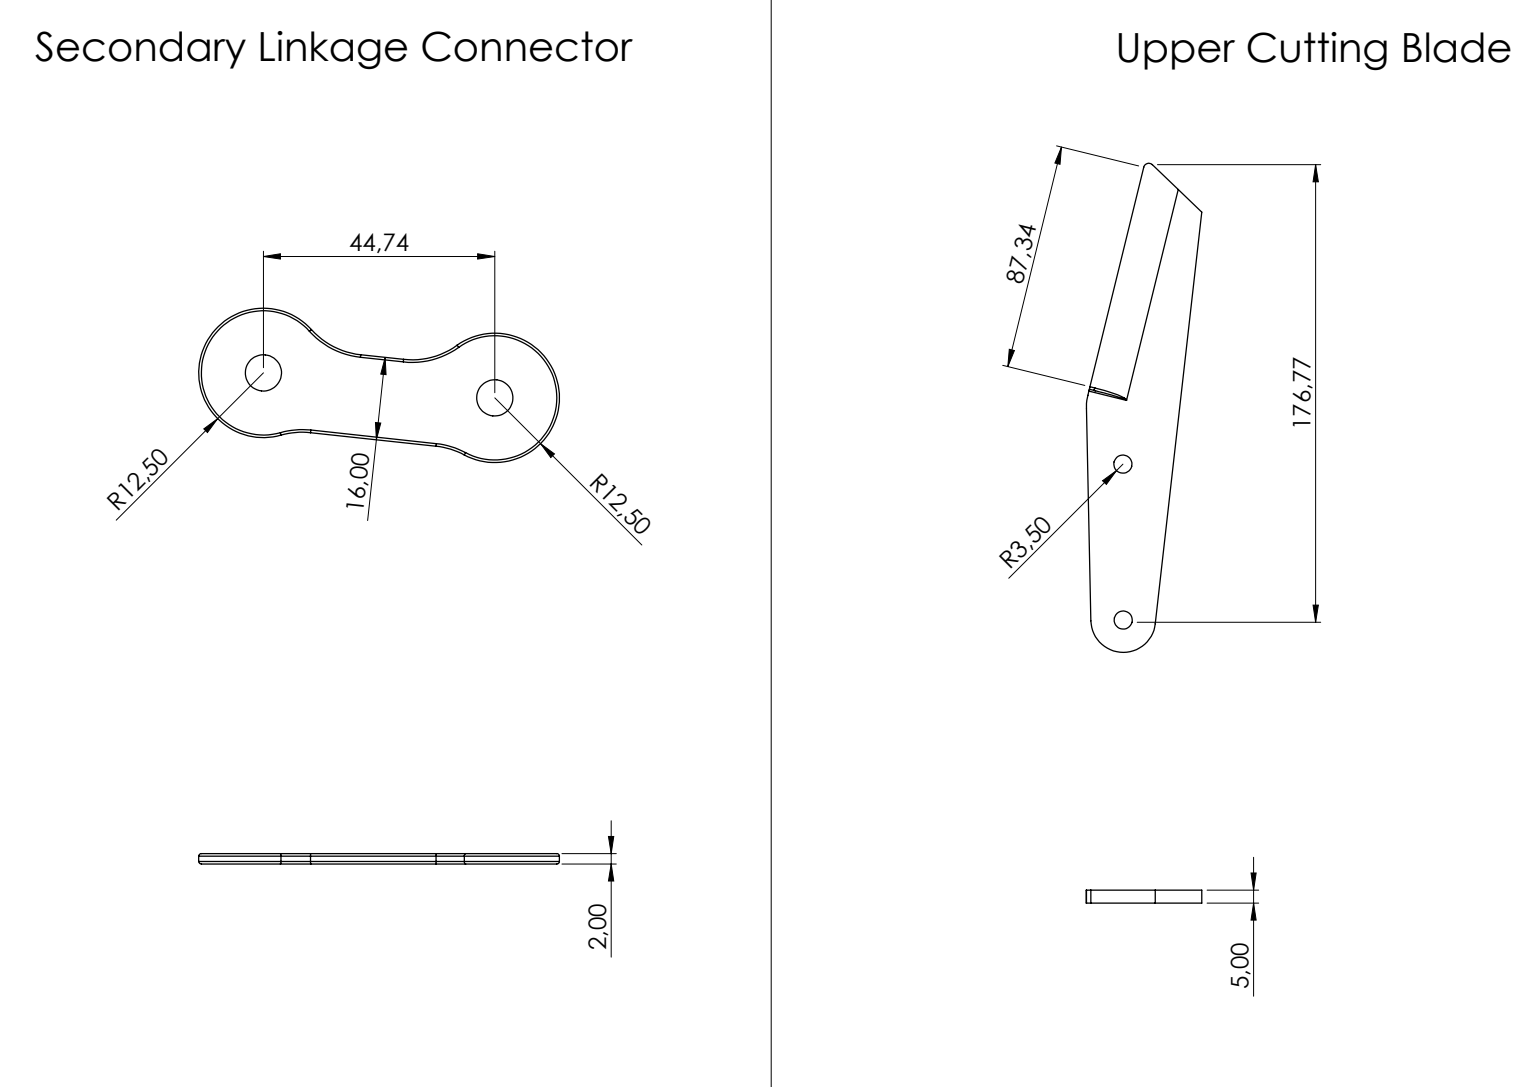
ISO-10303-21;
HEADER;
FILE_DESCRIPTION (('STEP AP214'),
    '1' );
FILE_NAME ('Upper Cutting Blade.step',
    '2026-10-06T08:24:18',
    ( '' ),
    ( '' ),
    'SwSTEP 2.0',
    'SolidWorks 2020',
    '' );
FILE_SCHEMA (( 'AUTOMOTIVE_DESIGN' ));
ENDSEC;

DATA;
#1=B_SPLINE_CURVE_WITH_KNOTS ( 'NONE', 3,
 ( #1947, #5214, #5583, #6285 ),
 .UNSPECIFIED., .F., .F.,
 ( 4, 4 ),
 ( 0.000000000000000000, 1.000000000000000000 ),
 .UNSPECIFIED. ) ;
#2=DIRECTION ( 'NONE',  ( -0.000000000000000000, 1.000000000000000000, 0.000000000000000000 ) ) ;
#8=CARTESIAN_POINT ( 'NONE',  ( -14.98500449093754483, -6.750000000000000000, -438.4247239981262396 ) ) ;
#9=CARTESIAN_POINT ( 'NONE',  ( -1.582652182125599660, -2.660653890702000091, -435.1382991101020821 ) ) ;
#16=CARTESIAN_POINT ( 'NONE',  ( -1.663986357696749074, -7.359447597713999478, -434.8428272099179708 ) ) ;
#37=DIRECTION ( 'NONE',  ( 0.000000000000000000, 1.000000000000000000, 0.000000000000000000 ) ) ;
#44=VECTOR ( 'NONE', #4470, 1000.000000000000114 ) ;
#64=LINE ( 'NONE', #8, #382 ) ;
#71=CARTESIAN_POINT ( 'NONE',  ( -0.1188650835482805701, -7.653137857774001240, -434.2605423690813495 ) ) ;
#78=VERTEX_POINT ( 'NONE', #124 ) ;
#81=CIRCLE ( 'NONE', #4200, 3.500000000000006217 ) ;
#89=CARTESIAN_POINT ( 'NONE',  ( -2.737771089256917811, -7.372713325221263325, -435.0800118814183861 ) ) ;
#97=CARTESIAN_POINT ( 'NONE',  ( -1.873948611767810357, -7.500000000000000000, -349.2478646809746579 ) ) ;
#115=CARTESIAN_POINT ( 'NONE',  ( -11.58158374908019894, -4.051769059165300391, -438.8373653579053553 ) ) ;
#117=DIRECTION ( 'NONE',  ( -0.2381566831044910626, 0.000000000000000000, 0.9712267471052612455 ) ) ;
#119=CARTESIAN_POINT ( 'NONE',  ( -0.6964476799210029823, -2.503143587811580861, -434.2208226102950448 ) ) ;
#124=CARTESIAN_POINT ( 'NONE',  ( -5.273242226636224217, -2.500000000000000000, -350.0814130718403590 ) ) ;
#127=CARTESIAN_POINT ( 'NONE',  ( 8.445486755484310493, -5.763031266960239485, -525.6917925150787596 ) ) ;
#129=CARTESIAN_POINT ( 'NONE',  ( -14.11853184716549059, -5.586257366442001882, -439.2418799830686567 ) ) ;
#131=ORIENTED_EDGE ( 'NONE', *, *, #4319, .T. ) ;
#138=EDGE_CURVE ( 'NONE', #9192, #3634, #10595, .T. ) ;
#140=AXIS2_PLACEMENT_3D ( 'NONE', #9839, #705, #3977 ) ;
#146=VERTEX_POINT ( 'NONE', #9795 ) ;
#152=ADVANCED_FACE ( 'NONE', ( #1627 ), #8180, .F. ) ;
#165=CARTESIAN_POINT ( 'NONE',  ( -3.785374802930533633, -3.175228950698999686, -436.5426513454903557 ) ) ;
#167=CYLINDRICAL_SURFACE ( 'NONE', #9611, 3.500000000000006217 ) ;
#170=CARTESIAN_POINT ( 'NONE',  ( -1.502676399155497666, -2.553500183759497055, -434.6331789313892386 ) ) ;
#174=CARTESIAN_POINT ( 'NONE',  ( -10.10557620461820783, -6.350202160722001388, -437.2724170503247478 ) ) ;
#176=CARTESIAN_POINT ( 'NONE',  ( -0.1242360338837507489, -2.350034431637000765, -434.3027510456794857 ) ) ;
#180=CARTESIAN_POINT ( 'NONE',  ( 8.029177897429777389, -4.293198024933910339, -525.7662775258050942 ) ) ;
#182=CARTESIAN_POINT ( 'NONE',  ( 8.590329508774594558, -5.782842335357056385, -525.6531578069093484 ) ) ;
#191=EDGE_LOOP ( 'NONE', ( #1720, #2254, #5403, #9051 ) ) ;
#202=ORIENTED_EDGE ( 'NONE', *, *, #2410, .F. ) ;
#208=( NAMED_UNIT ( * ) SI_UNIT ( $, .STERADIAN. ) SOLID_ANGLE_UNIT ( ) );
#234=CARTESIAN_POINT ( 'NONE',  ( 7.290921060855201752, -4.384180831252638910, -525.6208113643167508 ) ) ;
#236=CARTESIAN_POINT ( 'NONE',  ( 7.441233258528033190, -5.633901944276541229, -525.6643399796049607 ) ) ;
#238=DIRECTION ( 'NONE',  ( -0.2381557937579781570, -1.220925210680262645E-07, 0.9712269651834695150 ) ) ;
#250=CARTESIAN_POINT ( 'NONE',  ( -2.040571445035855636, -7.414593747479792718, -434.8398329727854730 ) ) ;
#253=EDGE_LOOP ( 'NONE', ( #1986, #2444 ) ) ;
#255=DIRECTION ( 'NONE',  ( -0.000000000000000000, 1.000000000000000000, 0.000000000000000000 ) ) ;
#276=CARTESIAN_POINT ( 'NONE',  ( -0.6583197226283303838, -2.500002886833834204, -434.1455329896276680 ) ) ;
#283=DIRECTION ( 'NONE',  ( -0.000000000000000000, 1.000000000000000000, 0.000000000000000000 ) ) ;
#287=CARTESIAN_POINT ( 'NONE',  ( 28.53863984632670636, -7.500000000000000000, -506.8274460463252353 ) ) ;
#302=DIRECTION ( 'NONE',  ( -0.000000000000000000, 1.000000000000000000, 0.000000000000000000 ) ) ;
#309=EDGE_CURVE ( 'NONE', #4938, #6833, #7633, .T. ) ;
#311=VECTOR ( 'NONE', #7522, 1000.000000000000114 ) ;
#312=B_SPLINE_CURVE_WITH_KNOTS ( 'NONE', 3,
 ( #4614, #3005, #5310, #9407, #7889, #6280, #1335, #5207, #2093, #7044, #1228, #5260, #3810, #10313, #5359, #7836, #485, #2950, #6223, #8534, #8486 ),
 .UNSPECIFIED., .F., .F.,
 ( 4, 1, 1, 1, 2, 2, 1, 1, 1, 1, 1, 1, 2, 2, 4 ),
 ( 0.000000000000000000, 0.2499999999999730771, 0.3749999999999595879, 0.4374999999999530931, 0.4687499999999498734, 0.4999999999999465983, 0.6249999999999374944, 0.6874999999999327205, 0.7187499999999277245, 0.7343749999999221734, 0.7421874999999192868, 0.7460937499999209521, 0.7480468749999217293, 0.7499999999999225064, 1.000000000000000000 ),
 .UNSPECIFIED. ) ;
#313=EDGE_CURVE ( 'NONE', #8716, #4497, #7817, .T. ) ;
#326=LINE ( 'NONE', #4560, #9098 ) ;
#327=DIRECTION ( 'NONE',  ( 0.000000000000000000, -1.000000000000000000, 0.000000000000000000 ) ) ;
#336=CARTESIAN_POINT ( 'NONE',  ( 7.538136778550191153, -5.645663747140947208, -525.6900796742911552 ) ) ;
#342=EDGE_CURVE ( 'NONE', #5251, #8235, #3736, .T. ) ;
#355=DIRECTION ( 'NONE',  ( -0.000000000000000000, 1.000000000000000000, 0.000000000000000000 ) ) ;
#362=CARTESIAN_POINT ( 'NONE',  ( -0.5452757643750816285, -7.478314948056999256, -434.2680375005485871 ) ) ;
#373=EDGE_CURVE ( 'NONE', #5743, #3634, #3350, .T. ) ;
#379=( BOUNDED_SURFACE ( )  B_SPLINE_SURFACE ( 3, 3, ( 
 ( #3396, #9259, #9950, #5161, #8434, #1074, #1023, #5853, #7635, #8489 ),
 ( #9144, #5053, #8334, #972, #4258, #7528, #174, #3449, #9205, #5106 ),
 ( #4309, #3504, #2902, #7046, #4459, #8641, #8536, #5261, #1178, #6121 ),
 ( #7891, #3812, #10155, #4565, #6282, #5361, #3653, #2151, #3007, #7099 ) ),
 .UNSPECIFIED., .F., .F., .T. ) 
 B_SPLINE_SURFACE_WITH_KNOTS ( ( 4, 4 ),
 ( 4, 1, 1, 1, 1, 1, 1, 4 ),
 ( 0.000000000000000000, 1.000000000000000000 ),
 ( 0.04004302100395999708, 0.1036559982346000053, 0.2203786577267000113, 0.3496747522196999580, 0.4912411616719999929, 0.6462853912813000257, 0.8150922079746999449, 0.8736421606905999671 ),
 .UNSPECIFIED. ) 
 GEOMETRIC_REPRESENTATION_ITEM ( )  RATIONAL_B_SPLINE_SURFACE ( (
 ( 1.237064798922000053, 1.237064798922000053, 1.237064798922000053, 1.237064798922000053, 1.237064798922000053, 1.237064798922000053, 1.237064798922000053, 1.237064798922000053, 1.237064798922000053, 1.237064798922000053),
 ( 0.9209784003594999602, 0.9209784003594999602, 0.9209784003594999602, 0.9209784003594999602, 0.9209784003594999602, 0.9209784003594999602, 0.9209784003594999602, 0.9209784003594999602, 0.9209784003594999602, 0.9209784003594999602),
 ( 0.9209784003594999602, 0.9209784003594999602, 0.9209784003594999602, 0.9209784003594999602, 0.9209784003594999602, 0.9209784003594999602, 0.9209784003594999602, 0.9209784003594999602, 0.9209784003594999602, 0.9209784003594999602),
 ( 1.237064798922000053, 1.237064798922000053, 1.237064798922000053, 1.237064798922000053, 1.237064798922000053, 1.237064798922000053, 1.237064798922000053, 1.237064798922000053, 1.237064798922000053, 1.237064798922000053) ) ) 
 REPRESENTATION_ITEM ( '' )  SURFACE ( )  );
#382=VECTOR ( 'NONE', #1674, 1000.000000000000114 ) ;
#385=CARTESIAN_POINT ( 'NONE',  ( 6.150179767644408990, -4.500000000000001776, -524.6161169473078871 ) ) ;
#386=DIRECTION ( 'NONE',  ( 0.9627070496199738869, -0.1321637200910051047, 0.2360675490272045596 ) ) ;
#400=DIRECTION ( 'NONE',  ( -0.9712267471052594692, 0.000000000000000000, -0.2381566831044984178 ) ) ;
#401=ORIENTED_EDGE ( 'NONE', *, *, #4319, .F. ) ;
#407=EDGE_CURVE ( 'NONE', #146, #5498, #4519, .T. ) ;
#409=CARTESIAN_POINT ( 'NONE',  ( -0.7256479603086914976, -7.501867437109999592, -434.1451055704292799 ) ) ;
#418=CARTESIAN_POINT ( 'NONE',  ( -0.6596894340221253206, -7.499999891561000886, -434.1397621899948263 ) ) ;
#429=CARTESIAN_POINT ( 'NONE',  ( -1.582652182125599660, -2.660653890702000091, -435.1382991101020821 ) ) ;
#435=B_SPLINE_CURVE_WITH_KNOTS ( 'NONE', 3,
 ( #4769, #8901, #8094, #8733, #8788, #10403, #10619, #2354, #4014, #790, #6372, #2295 ),
 .UNSPECIFIED., .F., .F.,
 ( 4, 2, 2, 2, 2, 4 ),
 ( 0.000000000000000000, 0.4999999999999995559, 0.7499999999999974465, 0.8749999999999965583, 0.9374999999999983347, 1.000000000000000000 ),
 .UNSPECIFIED. ) ;
#446=CARTESIAN_POINT ( 'NONE',  ( -0.6528312677253685914, -7.479800707286198502, -434.5251259939439024 ) ) ;
#454=CARTESIAN_POINT ( 'NONE',  ( 9.378959784071181360, -5.899999999999999467, -525.1866552614185366 ) ) ;
#464=CARTESIAN_POINT ( 'NONE',  ( -1.658294475769471310, -7.463038962712998270, -434.6370517716558197 ) ) ;
#475=CARTESIAN_POINT ( 'NONE',  ( -1.788249073448326953, -7.429140679109920598, -434.7441729133906279 ) ) ;
#483=DIRECTION ( 'NONE',  ( -0.000000000000000000, 1.000000000000000000, 0.000000000000000000 ) ) ;
#485=CARTESIAN_POINT ( 'NONE',  ( -3.771252382897392952, -2.975477256776445145, -436.1454489244006822 ) ) ;
#501=CARTESIAN_POINT ( 'NONE',  ( -0.5293798494821438938, -2.512522400030999137, -434.0497706731864582 ) ) ;
#519=DIRECTION ( 'NONE',  ( -0.000000000000000000, 1.000000000000000000, 0.000000000000000000 ) ) ;
#521=CARTESIAN_POINT ( 'NONE',  ( -0.9182485701526132971, -7.496877080320997422, -434.3056557713407528 ) ) ;
#526=ORIENTED_EDGE ( 'NONE', *, *, #7256, .F. ) ;
#550=CARTESIAN_POINT ( 'NONE',  ( -1.558284605000191947, -2.631303827346001878, -434.8033654657723446 ) ) ;
#556=DIRECTION ( 'NONE',  ( -0.000000000000000000, 1.000000000000000000, 0.000000000000000000 ) ) ;
#571=CARTESIAN_POINT ( 'NONE',  ( -0.1153702471463786128, -7.665106240334001342, -434.0348060233743581 ) ) ;
#574=VERTEX_POINT ( 'NONE', #5718 ) ;
#583=ORIENTED_EDGE ( 'NONE', *, *, #4956, .T. ) ;
#601=CIRCLE ( 'NONE', #6609, 3.500000000000006217 ) ;
#611=CARTESIAN_POINT ( 'NONE',  ( -1.837389479601686304, -2.655393054924001461, -434.9057872931240354 ) ) ;
#621=DIRECTION ( 'NONE',  ( -0.000000000000000000, 1.000000000000000000, 0.000000000000000000 ) ) ;
#629=CARTESIAN_POINT ( 'NONE',  ( -5.273242226636224217, -7.500000000000000000, -350.0814130718403590 ) ) ;
#637=ADVANCED_FACE ( 'NONE', ( #3830 ), #4049, .F. ) ;
#650=DIRECTION ( 'NONE',  ( -0.000000000000000000, 1.000000000000000000, 0.000000000000000000 ) ) ;
#655=ADVANCED_FACE ( 'NONE', ( #3024 ), #6350, .T. ) ;
#660=CARTESIAN_POINT ( 'NONE',  ( -1.444632214126728043, -2.659134901855999988, -434.9867182716628236 ) ) ;
#664=ORIENTED_EDGE ( 'NONE', *, *, #4434, .T. ) ;
#705=DIRECTION ( 'NONE',  ( -0.9712267471052612455, 0.000000000000000000, -0.2381566831044910626 ) ) ;
#714=CARTESIAN_POINT ( 'NONE',  ( -0.5380925645899466980, -2.513321162497997197, -434.0383604270527940 ) ) ;
#720=FACE_BOUND ( 'NONE', #6913, .T. ) ;
#722=VERTEX_POINT ( 'NONE', #8182 ) ;
#733=CARTESIAN_POINT ( 'NONE',  ( 9.378959784071181360, -5.899999999999999467, -525.1866552614185366 ) ) ;
#748=EDGE_LOOP ( 'NONE', ( #1545, #9667, #1018, #6857 ) ) ;
#752=CARTESIAN_POINT ( 'NONE',  ( -1.999999999997229772, -7.500000000000000000, -409.4999999999571969 ) ) ;
#759=CARTESIAN_POINT ( 'NONE',  ( -3.656057816511529168, -7.040919069177174805, -436.0988728614874503 ) ) ;
#770=EDGE_CURVE ( 'NONE', #2618, #5251, #7738, .T. ) ;
#771=CARTESIAN_POINT ( 'NONE',  ( -1.000888714456147133, -7.421678258158998176, -434.5721179219322039 ) ) ;
#790=CARTESIAN_POINT ( 'NONE',  ( -2.272356604769890431, -2.599354866276060605, -434.9211891149597591 ) ) ;
#805=DIRECTION ( 'NONE',  ( -0.9712267471052594692, 0.000000000000000000, -0.2381566831044984178 ) ) ;
#815=CARTESIAN_POINT ( 'NONE',  ( -15.03660170392436335, -3.530928676948000167, -439.4670019462156461 ) ) ;
#822=CARTESIAN_POINT ( 'NONE',  ( -0.3462645226701464574, -7.523938431909999558, -434.3437067901672322 ) ) ;
#824=CARTESIAN_POINT ( 'NONE',  ( -0.6228901166779408083, -2.499999376604999934, -434.1632067468180480 ) ) ;
#840=ORIENTED_EDGE ( 'NONE', *, *, #770, .T. ) ;
#856=CARTESIAN_POINT ( 'NONE',  ( -13.22841709878402483, -6.750000000003000267, -437.9939892205655383 ) ) ;
#869=CARTESIAN_POINT ( 'NONE',  ( -1.322461528884503412, -7.357049826291000905, -434.9394999171997824 ) ) ;
#880=EDGE_CURVE ( 'NONE', #5498, #146, #2568, .T. ) ;
#890=VERTEX_POINT ( 'NONE', #6702 ) ;
#907=ORIENTED_EDGE ( 'NONE', *, *, #4640, .T. ) ;
#908=CARTESIAN_POINT ( 'NONE',  ( -5.874649674696526880, -3.342435975618997634, -436.3259412683626692 ) ) ;
#922=CARTESIAN_POINT ( 'NONE',  ( -0.9319947458880994962, -7.428963293140000701, -434.5389931698585428 ) ) ;
#943=ORIENTED_EDGE ( 'NONE', *, *, #3912, .F. ) ;
#965=CARTESIAN_POINT ( 'NONE',  ( -11.73517431002995970, -4.202811174509099246, -438.1641048472901616 ) ) ;
#972=CARTESIAN_POINT ( 'NONE',  ( -4.039076881902885496, -6.821318530964001425, -435.8791522177131696 ) ) ;
#979=CARTESIAN_POINT ( 'NONE',  ( 8.820893615063965854, -5.815056166419472206, -525.5682599993908752 ) ) ;
#1002=B_SPLINE_CURVE_WITH_KNOTS ( 'NONE', 3,
 ( #4633, #7160, #7904, #10431, #2110, #3071, #6345, #4521, #7110, #6511, #9846, #5753, #8178, #7372, #9039, #4045, #8278, #2536, #4949, #4849, #2484 ),
 .UNSPECIFIED., .F., .F.,
 ( 4, 1, 1, 1, 2, 2, 2, 2, 1, 1, 2, 2, 4 ),
 ( 0.000000000000000000, 0.1249999999994945710, 0.1874999999991950606, 0.2187499999990910604, 0.2343749999990832888, 0.2499999999990755173, 0.3749999999992109090, 0.4999999999993463007, 0.6249999999994816369, 0.6874999999995808908, 0.7187499999996315170, 0.7499999999996821431, 1.000000000000000000 ),
 .UNSPECIFIED. ) ;
#1005=CARTESIAN_POINT ( 'NONE',  ( -16.11962419174959393, -2.500000000000000000, -430.9361393731155658 ) ) ;
#1014=CARTESIAN_POINT ( 'NONE',  ( -4.040158012961684086, -3.178778163799998779, -435.8794274319448050 ) ) ;
#1018=ORIENTED_EDGE ( 'NONE', *, *, #5034, .F. ) ;
#1022=SURFACE_SIDE_STYLE ('',( #6726 ) ) ;
#1023=CARTESIAN_POINT ( 'NONE',  ( -10.21689005072306422, -7.047891920729001392, -437.2157279943754133 ) ) ;
#1029=CARTESIAN_POINT ( 'NONE',  ( 8.337581009124432896, -4.251569741560065729, -525.7130236167810153 ) ) ;
#1030=CARTESIAN_POINT ( 'NONE',  ( -1.327990674002025528, -7.383908396211002589, -435.1679363805569665 ) ) ;
#1045=( BOUNDED_CURVE ( )  B_SPLINE_CURVE ( 3, ( #9621, #4574, #8700, #6128 ),
 .UNSPECIFIED., .F., .F. ) 
 B_SPLINE_CURVE_WITH_KNOTS ( ( 4, 4 ),
 ( 0.000000000000000000, 1.000000000000000000 ),
 .UNSPECIFIED. ) 
 CURVE ( )  GEOMETRIC_REPRESENTATION_ITEM ( )  RATIONAL_B_SPLINE_CURVE ( ( 1.017160811567055401, 0.9969340269212683125, 0.9945876386442641381, 1.010121646736042766 ) ) 
 REPRESENTATION_ITEM ( '' )  );
#1069=CARTESIAN_POINT ( 'NONE',  ( -1.437615631311345288, -2.692042927306998568, -435.8453383182137486 ) ) ;
#1072=CARTESIAN_POINT ( 'NONE',  ( -0.9894400438770221129, -2.521929977679939316, -434.4064049843834141 ) ) ;
#1074=CARTESIAN_POINT ( 'NONE',  ( -8.039695956235750174, -7.171008361171001155, -436.6144689615417747 ) ) ;
#1088=ORIENTED_EDGE ( 'NONE', *, *, #313, .F. ) ;
#1100=ORIENTED_EDGE ( 'NONE', *, *, #6861, .T. ) ;
#1110=CIRCLE ( 'NONE', #2316, 0.7499999999999997780 ) ;
#1114=CARTESIAN_POINT ( 'NONE',  ( -0.9643324756131976816, -7.495094651894998350, -434.3305354681787662 ) ) ;
#1121=ORIENTED_EDGE ( 'NONE', *, *, #9520, .F. ) ;
#1136=DIRECTION ( 'NONE',  ( 0.000000000000000000, -1.000000000000000000, -0.000000000000000000 ) ) ;
#1139=DIRECTION ( 'NONE',  ( -0.9627072696281171460, 0.1321637200910011078, -0.2360666518102109701 ) ) ;
#1159=B_SPLINE_CURVE_WITH_KNOTS ( 'NONE', 3,
 ( #4416, #8440, #10011, #3561, #979, #5920, #182, #6678, #127, #8392, #9369, #2003, #10113, #9958, #5860, #7693, #7587, #1949, #2753, #336, #4211, #3404, #5115, #3613, #1843, #236, #3456, #5060, #5267, #4370, #9315 ),
 .UNSPECIFIED., .F., .F.,
 ( 4, 2, 2, 2, 1, 1, 1, 2, 2, 2, 2, 1, 1, 1, 1, 2, 2, 2, 4 ),
 ( 0.000000000000000000, 0.1250000000002775280, 0.1875000000004162504, 0.2187500000004856116, 0.2343750000005130896, 0.2421875000005322132, 0.2460937500005417611, 0.2480468750005504208, 0.2500000000005591083, 0.3750000000010509371, 0.4375000000012961299, 0.4687500000014282464, 0.4843750000015074053, 0.4921875000015624169, 0.4960937500015898949, 0.4980468750016032176, 0.5000000000016164847, 0.7500000000008082424, 1.000000000000000000 ),
 .UNSPECIFIED. ) ;
#1163=CARTESIAN_POINT ( 'NONE',  ( -0.8117387980152629412, -7.500462190812000607, -434.2418354198644010 ) ) ;
#1178=CARTESIAN_POINT ( 'NONE',  ( -12.82600522015554922, -5.696851206212700802, -438.3416979569461205 ) ) ;
#1181=FACE_OUTER_BOUND ( 'NONE', #6826, .T. ) ;
#1184=AXIS2_PLACEMENT_3D ( 'NONE', #97, #5779, #6762 ) ;
#1208=CARTESIAN_POINT ( 'NONE',  ( 6.052780067456072999, -4.500000000000000888, -524.2189112390747141 ) ) ;
#1212=FILL_AREA_STYLE_COLOUR ( '', #7652 ) ;
#1222=DIRECTION ( 'NONE',  ( -0.9712267471052611345, 0.000000000000000000, -0.2381566831044912569 ) ) ;
#1228=CARTESIAN_POINT ( 'NONE',  ( -4.443194270446590544, -3.070841006776869886, -436.4083858720387639 ) ) ;
#1236=ORIENTED_EDGE ( 'NONE', *, *, #6395, .F. ) ;
#1238=LINE ( 'NONE', #9569, #7592 ) ;
#1253=ORIENTED_EDGE ( 'NONE', *, *, #1527, .F. ) ;
#1263=ORIENTED_EDGE ( 'NONE', *, *, #3216, .T. ) ;
#1264=STYLED_ITEM ( 'NONE', ( #2643 ), #8937 ) ;
#1274=CARTESIAN_POINT ( 'NONE',  ( -1.249129537600907502, -7.462014900586536825, -434.5271252024986666 ) ) ;
#1291=ADVANCED_FACE ( 'NONE', ( #1181 ), #10221, .T. ) ;
#1300=CARTESIAN_POINT ( 'NONE',  ( -0.6576834034345514501, -2.538582342225996769, -434.3791788602677570 ) ) ;
#1309=CARTESIAN_POINT ( 'NONE',  ( -4.134979495079278422, -6.972766829544778666, -436.2920240787863690 ) ) ;
#1310=CARTESIAN_POINT ( 'NONE',  ( -14.74684780783305449, -4.500000000000000888, -439.3959507452315165 ) ) ;
#1326=B_SPLINE_CURVE_WITH_KNOTS ( 'NONE', 3,
 ( #429, #10262, #8638, #3605 ),
 .UNSPECIFIED., .F., .F.,
 ( 4, 4 ),
 ( 0.000000000000000000, 1.000000000000000000 ),
 .UNSPECIFIED. ) ;
#1332=CARTESIAN_POINT ( 'NONE',  ( 19.38368284813939013, -2.500000000000000000, -515.5999187775453265 ) ) ;
#1335=CARTESIAN_POINT ( 'NONE',  ( -6.619999202174732034, -3.376841163498135234, -437.1676759332182769 ) ) ;
#1338=EDGE_CURVE ( 'NONE', #5915, #6684, #1, .T. ) ;
#1343=CARTESIAN_POINT ( 'NONE',  ( 6.052780067456072999, -4.500000000000000888, -524.2189112390747141 ) ) ;
#1352=CARTESIAN_POINT ( 'NONE',  ( -0.8844900259107285612, -2.565904207356001443, -434.5153608183709935 ) ) ;
#1353=ORIENTED_EDGE ( 'NONE', *, *, #7256, .T. ) ;
#1365=ORIENTED_EDGE ( 'NONE', *, *, #5468, .F. ) ;
#1370=CARTESIAN_POINT ( 'NONE',  ( -1.547234103168566133, -7.369705175477000658, -434.7990518850289163 ) ) ;
#1390=ORIENTED_EDGE ( 'NONE', *, *, #4717, .F. ) ;
#1391=DIRECTION ( 'NONE',  ( -0.9712267471052594692, 0.000000000000000000, -0.2381566831044984178 ) ) ;
#1406=CARTESIAN_POINT ( 'NONE',  ( -0.7175256489034935736, -2.498213111830998923, -434.1510992972750387 ) ) ;
#1419=FACE_OUTER_BOUND ( 'NONE', #4482, .T. ) ;
#1435=CARTESIAN_POINT ( 'NONE',  ( -15.16362200326591569, -7.500000000000000000, -437.6963039377973246 ) ) ;
#1444=CARTESIAN_POINT ( 'NONE',  ( -14.78164251960286890, -4.500000000000000000, -439.2540544344155933 ) ) ;
#1450=CLOSED_SHELL ( 'NONE', ( #6125, #6680, #4249, #152, #2598, #9705, #4681, #8027, #2131, #1291, #655, #6920, #4479, #4185, #3013, #3240, #637, #5572, #6836, #2413, #2799, #2213, #8047, #6176, #7498 ) ) ;
#1454=EDGE_CURVE ( 'NONE', #7492, #9535, #2957, .T. ) ;
#1466=CARTESIAN_POINT ( 'NONE',  ( -0.5984921290374501934, -2.530241314762997629, -434.3301463708660322 ) ) ;
#1473=CARTESIAN_POINT ( 'NONE',  ( -0.5534908175310586653, -2.500000333914000006, -434.2941325283891274 ) ) ;
#1502=CARTESIAN_POINT ( 'NONE',  ( -14.85178883355849599, -4.396734861472281430, -438.9679907580307940 ) ) ;
#1504=ORIENTED_EDGE ( 'NONE', *, *, #2729, .T. ) ;
#1506=PRODUCT_DEFINITION_SHAPE ( 'NONE', 'NONE',  #2191 ) ;
#1518=CARTESIAN_POINT ( 'NONE',  ( -1.668977462971013681, -2.537472099014000726, -434.6413441610087034 ) ) ;
#1521=DIRECTION ( 'NONE',  ( -0.000000000000000000, 1.000000000000000000, 0.000000000000000000 ) ) ;
#1527=EDGE_CURVE ( 'NONE', #9271, #890, #5926, .T. ) ;
#1528=EDGE_LOOP ( 'NONE', ( #5275, #7312, #1559, #3644, #3139, #4760, #5881, #4377, #9229 ) ) ;
#1530=VERTEX_POINT ( 'NONE', #5273 ) ;
#1545=ORIENTED_EDGE ( 'NONE', *, *, #9391, .T. ) ;
#1559=ORIENTED_EDGE ( 'NONE', *, *, #4277, .T. ) ;
#1576=CARTESIAN_POINT ( 'NONE',  ( -0.1454145850583489497, -8.513384478312998382, -435.8155006440865691 ) ) ;
#1580=CARTESIAN_POINT ( 'NONE',  ( -0.4619277171041915042, -7.556499546952999857, -434.7365042083650906 ) ) ;
#1582=DIRECTION ( 'NONE',  ( -0.9712267471052612455, 0.000000000000000000, -0.2381566831044910626 ) ) ;
#1583=FACE_OUTER_BOUND ( 'NONE', #10228, .T. ) ;
#1592=AXIS2_PLACEMENT_3D ( 'NONE', #4702, #621, #6470 ) ;
#1599=ORIENTED_EDGE ( 'NONE', *, *, #3133, .T. ) ;
#1626=CARTESIAN_POINT ( 'NONE',  ( -1.486103177728019809, -2.642483842335999089, -435.2287432255328667 ) ) ;
#1627=FACE_OUTER_BOUND ( 'NONE', #4357, .T. ) ;
#1633=CARTESIAN_POINT ( 'NONE',  ( -0.5253760780244931539, -7.541458695310001126, -434.7805624543377689 ) ) ;
#1639=ORIENTED_EDGE ( 'NONE', *, *, #5745, .F. ) ;
#1644=DIRECTION ( 'NONE',  ( 0.9936574763089274231, 0.000000000000000000, 0.1124491875265153373 ) ) ;
#1663=ORIENTED_EDGE ( 'NONE', *, *, #407, .T. ) ;
#1674=DIRECTION ( 'NONE',  ( 0.9712269959794516128, -1.472254293302932272E-12, 0.2381556681683856258 ) ) ;
#1682=EDGE_CURVE ( 'NONE', #9271, #722, #5114, .T. ) ;
#1683=CARTESIAN_POINT ( 'NONE',  ( -0.1066158053962373981, -7.660711547938000798, -434.1593156514779253 ) ) ;
#1696=PLANE ( 'NONE',  #3521 ) ;
#1720=ORIENTED_EDGE ( 'NONE', *, *, #1454, .F. ) ;
#1722=CARTESIAN_POINT ( 'NONE',  ( -1.723815153757401353, -2.911508528774001459, -435.2348705281305001 ) ) ;
#1728=CARTESIAN_POINT ( 'NONE',  ( -0.6577138333327989805, -2.500183709831155454, -434.1612907480973149 ) ) ;
#1735=CARTESIAN_POINT ( 'NONE',  ( -1.121771287418490415, -7.384865809656000479, -434.8579640789354244 ) ) ;
#1748=CARTESIAN_POINT ( 'NONE',  ( -1.813125098999968543, -7.427867185880000278, -434.7536662776001322 ) ) ;
#1754=ORIENTED_EDGE ( 'NONE', *, *, #3459, .T. ) ;
#1759=EDGE_CURVE ( 'NONE', #6366, #4799, #1002, .T. ) ;
#1760=LINE ( 'NONE', #9929, #4624 ) ;
#1775=FACE_OUTER_BOUND ( 'NONE', #748, .T. ) ;
#1780=CARTESIAN_POINT ( 'NONE',  ( -0.6695406252879771980, -2.501212138556309306, -434.1886289273209627 ) ) ;
#1785=CARTESIAN_POINT ( 'NONE',  ( -0.1791381520249625270, -2.339610688496001512, -433.8702690752436411 ) ) ;
#1790=CARTESIAN_POINT ( 'NONE',  ( -1.009071087474297190, -7.440846336948001571, -435.0353261705186583 ) ) ;
#1803=DIRECTION ( 'NONE',  ( -0.000000000000000000, 1.000000000000000000, 0.000000000000000000 ) ) ;
#1821=( NAMED_UNIT ( * ) PLANE_ANGLE_UNIT ( ) SI_UNIT ( $, .RADIAN. ) );
#1833=LINE ( 'NONE', #856, #311 ) ;
#1842=CARTESIAN_POINT ( 'NONE',  ( 9.378959784071181360, -4.100000000000000533, -525.1866552614185366 ) ) ;
#1843=CARTESIAN_POINT ( 'NONE',  ( 7.441755802380456863, -5.633964924930761065, -525.6644890118283229 ) ) ;
#1870=EDGE_LOOP ( 'NONE', ( #10144, #6393 ) ) ;
#1882=CARTESIAN_POINT ( 'NONE',  ( -12.67186291068377102, -4.210876960398400648, -439.0233713709748145 ) ) ;
#1886=CIRCLE ( 'NONE', #4802, 1.000010080120980804 ) ;
#1896=CARTESIAN_POINT ( 'NONE',  ( 6.760923308610696125, -4.443194654328453730, -525.3178833974152440 ) ) ;
#1898=CARTESIAN_POINT ( 'NONE',  ( -12.86189863199293093, -5.758762107780500017, -438.9337381413729418 ) ) ;
#1917=FACE_OUTER_BOUND ( 'NONE', #7814, .T. ) ;
#1927=LINE ( 'NONE', #7567, #7093 ) ;
#1936=CARTESIAN_POINT ( 'NONE',  ( -13.08309215884270138, -3.120241701627000985, -437.9645355315274173 ) ) ;
#1941=( NAMED_UNIT ( * ) PLANE_ANGLE_UNIT ( ) SI_UNIT ( $, .RADIAN. ) );
#1947=CARTESIAN_POINT ( 'NONE',  ( -1.813125407131493949, -2.572135581867000198, -434.7536649739391237 ) ) ;
#1948=FACE_BOUND ( 'NONE', #10054, .T. ) ;
#1949=CARTESIAN_POINT ( 'NONE',  ( 7.681427628432651922, -5.663384406618502176, -525.7189183918870867 ) ) ;
#1952=EDGE_CURVE ( 'NONE', #8193, #5743, #2223, .T. ) ;
#1957=ORIENTED_EDGE ( 'NONE', *, *, #4434, .F. ) ;
#1968=CYLINDRICAL_SURFACE ( 'NONE', #9194, 0.7499999999999997780 ) ;
#1977=CARTESIAN_POINT ( 'NONE',  ( -0.5023555725018206131, -7.489090630217000388, -434.1119911457818716 ) ) ;
#1985=LINE ( 'NONE', #2188, #10502 ) ;
#1986=ORIENTED_EDGE ( 'NONE', *, *, #3319, .T. ) ;
#1987=CARTESIAN_POINT ( 'NONE',  ( -0.6780083913994491285, -7.498182470000450017, -434.1985855385974560 ) ) ;
#2003=CARTESIAN_POINT ( 'NONE',  ( 8.342417508530179049, -5.749081105070941611, -525.7122382318706286 ) ) ;
#2009=DIRECTION ( 'NONE',  ( 0.2381566831044910626, 0.000000000000000000, -0.9712267471052612455 ) ) ;
#2019=ORIENTED_EDGE ( 'NONE', *, *, #4921, .T. ) ;
#2025=CARTESIAN_POINT ( 'NONE',  ( -1.873948611767810357, -7.500000000000000000, -349.2478646809746579 ) ) ;
#2027=CARTESIAN_POINT ( 'NONE',  ( -0.5174164570134516250, -7.488494838810996868, -434.0682185966899169 ) ) ;
#2032=ORIENTED_EDGE ( 'NONE', *, *, #3049, .T. ) ;
#2057=LINE ( 'NONE', #6086, #10332 ) ;
#2071=DIRECTION ( 'NONE',  ( 0.6918631112021627061, 0.000000000000000000, -0.7220286942758327164 ) ) ;
#2076=CARTESIAN_POINT ( 'NONE',  ( -0.7865748771364371450, -7.501119061185001158, -434.2245970632208127 ) ) ;
#2087=CARTESIAN_POINT ( 'NONE',  ( -15.34933947562448076, -6.750000000000000000, -437.7418441346085274 ) ) ;
#2093=CARTESIAN_POINT ( 'NONE',  ( -5.875275055693564674, -3.272594625989450723, -436.9218166935183376 ) ) ;
#2099=DIRECTION ( 'NONE',  ( -0.2381566831044918675, 0.000000000000000000, 0.9712267471052610235 ) ) ;
#2110=CARTESIAN_POINT ( 'NONE',  ( -14.83150119643293330, -5.565240525586856002, -439.0507257690958909 ) ) ;
#2112=ORIENTED_EDGE ( 'NONE', *, *, #2260, .T. ) ;
#2129=MECHANICAL_DESIGN_GEOMETRIC_PRESENTATION_REPRESENTATION('',(#1264),#10532);
#2130=CARTESIAN_POINT ( 'NONE',  ( -1.284201520726217627, -7.481087858561002335, -434.4823192484363403 ) ) ;
#2131=ADVANCED_FACE ( 'NONE', ( #8935 ), #5707, .T. ) ;
#2151=CARTESIAN_POINT ( 'NONE',  ( -11.57898025333339831, -5.948622255021098759, -438.8369007677023319 ) ) ;
#2165=CARTESIAN_POINT ( 'NONE',  ( -0.4139159552628927652, -2.492503281179000663, -434.4399094585419903 ) ) ;
#2181=CARTESIAN_POINT ( 'NONE',  ( -1.552911365449734626, -7.327055393686999984, -435.0269566445958276 ) ) ;
#2188=CARTESIAN_POINT ( 'NONE',  ( -14.98500449093754483, -6.508849730028000380, -438.4247239981262396 ) ) ;
#2190=CARTESIAN_POINT ( 'NONE',  ( -1.099124599181354522, -7.471261185735560417, -434.4594340131810100 ) ) ;
#2191=PRODUCT_DEFINITION ( 'UNKNOWN', '', #5412, #7223 ) ;
#2213=ADVANCED_FACE ( 'NONE', ( #1948, #9905, #2651 ), #3510, .T. ) ;
#2218=CARTESIAN_POINT ( 'NONE',  ( -0.3413170418743253776, -2.457820343117000039, -433.9546262319294669 ) ) ;
#2223=LINE ( 'NONE', #6352, #6367 ) ;
#2241=ORIENTED_EDGE ( 'NONE', *, *, #6861, .F. ) ;
#2254=ORIENTED_EDGE ( 'NONE', *, *, #9718, .F. ) ;
#2260=EDGE_CURVE ( 'NONE', #5868, #10390, #7313, .T. ) ;
#2270=CARTESIAN_POINT ( 'NONE',  ( -1.170915164613087756, -2.622174536531001188, -434.8787092738958791 ) ) ;
#2274=ORIENTED_EDGE ( 'NONE', *, *, #5034, .T. ) ;
#2278=UNCERTAINTY_MEASURE_WITH_UNIT (LENGTH_MEASURE( 1.000000000000000082E-05 ), #10040, 'distance_accuracy_value', 'NONE');
#2295=CARTESIAN_POINT ( 'NONE',  ( -1.813125407131493949, -2.572135581867000198, -434.7536649739391237 ) ) ;
#2304=CARTESIAN_POINT ( 'NONE',  ( -15.54870946350325767, -7.500000000000000000, -436.1258788022018393 ) ) ;
#2315=CYLINDRICAL_SURFACE ( 'NONE', #3737, 3.500000000000006217 ) ;
#2316=AXIS2_PLACEMENT_3D ( 'NONE', #7503, #9874, #37 ) ;
#2326=CARTESIAN_POINT ( 'NONE',  ( -1.897969053490322855, -2.548986172702000896, -434.7293254325074940 ) ) ;
#2333=VERTEX_POINT ( 'NONE', #2805 ) ;
#2345=B_SPLINE_CURVE_WITH_KNOTS ( 'NONE', 3,
 ( #1748, #250, #9010, #89, #8197, #5824, #3366, #6643, #9918, #2555, #9116, #10178 ),
 .UNSPECIFIED., .F., .F.,
 ( 4, 2, 2, 2, 2, 4 ),
 ( 0.000000000000000000, 0.06249999999999888978, 0.1249999999999977796, 0.2499999999999998890, 0.4999999999999998890, 1.000000000000000000 ),
 .UNSPECIFIED. ) ;
#2354=CARTESIAN_POINT ( 'NONE',  ( -2.971092673426039443, -2.641283117323076191, -435.1576634133632524 ) ) ;
#2364=B_SPLINE_CURVE_WITH_KNOTS ( 'NONE', 3,
 ( #8051, #7252, #5630, #3921, #3869, #8746, #5578, #4027, #4081, #8860, #7146, #10579, #10520, #1502, #4784, #3222, #1444, #6384 ),
 .UNSPECIFIED., .F., .F.,
 ( 4, 1, 1, 1, 1, 2, 2, 1, 1, 2, 2, 4 ),
 ( 0.000000000000000000, 0.2499999999994746425, 0.3749999999992318367, 0.4374999999991385780, 0.4687499999990925592, 0.4843749999990695221, 0.4999999999990465405, 0.6249999999991870947, 0.6874999999993030020, 0.7187499999993127719, 0.7499999999993226529, 1.000000000000000000 ),
 .UNSPECIFIED. ) ;
#2367=CARTESIAN_POINT ( 'NONE',  ( -1.873948611767810357, -2.500000000000000000, -349.2478646809746579 ) ) ;
#2378=CARTESIAN_POINT ( 'NONE',  ( -2.975649281827347448, -7.138022370016234852, -435.8156820327864693 ) ) ;
#2380=CARTESIAN_POINT ( 'NONE',  ( -0.8018440996563184209, -2.556536707011997311, -434.4710415144371041 ) ) ;
#2385=CARTESIAN_POINT ( 'NONE',  ( -0.3206729354815163191, -7.530925261025000594, -434.2912207255791373 ) ) ;
#2393=ORIENTED_EDGE ( 'NONE', *, *, #3216, .F. ) ;
#2410=EDGE_CURVE ( 'NONE', #4588, #6311, #9403, .T. ) ;
#2413=ADVANCED_FACE ( 'NONE', ( #6394 ), #2315, .F. ) ;
#2429=CARTESIAN_POINT ( 'NONE',  ( -3.355145859302810507, -7.083804960661745476, -435.9754648412450138 ) ) ;
#2438=CARTESIAN_POINT ( 'NONE',  ( -0.1525530514593775588, -7.663337276471000159, -433.9190241679935411 ) ) ;
#2440=CARTESIAN_POINT ( 'NONE',  ( -0.5691333845031163463, -2.499999797932000334, -434.2421446687361026 ) ) ;
#2444=ORIENTED_EDGE ( 'NONE', *, *, #9718, .T. ) ;
#2450=FACE_OUTER_BOUND ( 'NONE', #7648, .T. ) ;
#2468=FACE_OUTER_BOUND ( 'NONE', #6148, .T. ) ;
#2484=CARTESIAN_POINT ( 'NONE',  ( -14.98500449093754483, -6.508849730028000380, -438.4247239981262396 ) ) ;
#2490=VECTOR ( 'NONE', #4188, 1000.000000000000000 ) ;
#2494=CARTESIAN_POINT ( 'NONE',  ( -1.219008076252173778, -7.371161895518000939, -434.8982261995575413 ) ) ;
#2528=CARTESIAN_POINT ( 'NONE',  ( -2.038789940206844342, -2.521785824191000280, -434.7311834052255790 ) ) ;
#2532=CARTESIAN_POINT ( 'NONE',  ( -1.743229001746446682, -2.568129413088056978, -434.7271494043006896 ) ) ;
#2536=CARTESIAN_POINT ( 'NONE',  ( -14.96226901326146042, -6.078566365972378982, -438.5174415475119076 ) ) ;
#2537=CARTESIAN_POINT ( 'NONE',  ( -0.5141583095772008782, -2.456010981267997551, -434.7739004999450003 ) ) ;
#2541=CARTESIAN_POINT ( 'NONE',  ( 8.369319885711609786, -4.247274070869474727, -525.7071792109185253 ) ) ;
#2543=CARTESIAN_POINT ( 'NONE',  ( -1.730441907225505727, -7.305146192242999881, -435.0908526137575905 ) ) ;
#2555=CARTESIAN_POINT ( 'NONE',  ( -9.379641673262440804, -6.977332597345990095, -437.0255175026235293 ) ) ;
#2558=ORIENTED_EDGE ( 'NONE', *, *, #4956, .F. ) ;
#2559=CARTESIAN_POINT ( 'NONE',  ( -0.6233307549567066452, -7.499999885133000532, -434.1629327817910280 ) ) ;
#2568=CIRCLE ( 'NONE', #1184, 3.500000000000006217 ) ;
#2581=( BOUNDED_CURVE ( )  B_SPLINE_CURVE ( 3, ( #7578, #9947, #2532, #7421, #170, #5965, #6014, #8332, #9091, #1072, #2642, #3447, #10002, #4358, #119, #1780, #1728, #276, #8222 ),
 .UNSPECIFIED., .F., .T. ) 
 B_SPLINE_CURVE_WITH_KNOTS ( ( 4, 1, 1, 1, 1, 1, 1, 1, 1, 1, 1, 1, 1, 1, 1, 1, 4 ),
 ( 0.000000000000000000, 0.02240047936246757077, 0.1327950495784611662, 0.2340085511830341525, 0.3267384236920149454, 0.4118026492331378074, 0.4900892306436237522, 0.5625168287438816472, 0.6299155825606346237, 0.6928641569844152803, 0.7516748739333113383, 0.8063000023450603848, 0.8556381163399817691, 0.8990751865928527931, 0.9381911258101325313, 0.9762570717716427815, 1.000000000000000000 ),
 .UNSPECIFIED. ) 
 CURVE ( )  GEOMETRIC_REPRESENTATION_ITEM ( )  RATIONAL_B_SPLINE_CURVE ( ( 1.017164269003578481, 1.017164269003578481, 1.017164269003578481, 1.017164269003578481, 1.017164269003578481, 1.017164269003578481, 1.017164269003578481, 1.017164269003578481, 1.017164269003578481, 1.017164269003578481, 1.017164269003578481, 1.017164269003578481, 1.017164269003578481, 1.017164269003578481, 1.017164269003578481, 1.017164269003578481, 1.017164269003578481, 1.017164269003578481, 1.017164269003578481 ) ) 
 REPRESENTATION_ITEM ( '' )  );
#2582=CARTESIAN_POINT ( 'NONE',  ( -1.093371887104504614, -1.934387371788998111, -435.9299591300448924 ) ) ;
#2596=EDGE_CURVE ( 'NONE', #9045, #4799, #1833, .T. ) ;
#2597=CARTESIAN_POINT ( 'NONE',  ( 7.733184489064065303, -4.330975896438657102, -525.7488827635337429 ) ) ;
#2598=ADVANCED_FACE ( 'NONE', ( #1775 ), #6545, .F. ) ;
#2601=CARTESIAN_POINT ( 'NONE',  ( -12.99025672594594027, -3.249999999996000088, -438.9652310147267826 ) ) ;
#2618=VERTEX_POINT ( 'NONE', #6777 ) ;
#2619=CIRCLE ( 'NONE', #6036, 20.00000000000000355 ) ;
#2628=AXIS2_PLACEMENT_3D ( 'NONE', #7742, #6231, #386 ) ;
#2637=CARTESIAN_POINT ( 'NONE',  ( -7.895874901503558085, -3.499933318827000317, -436.7910735983360269 ) ) ;
#2642=CARTESIAN_POINT ( 'NONE',  ( -0.9130074951844157072, -2.517145578169100339, -434.3665436561622641 ) ) ;
#2643=PRESENTATION_STYLE_ASSIGNMENT (( #6621 ) ) ;
#2651=FACE_OUTER_BOUND ( 'NONE', #1528, .T. ) ;
#2652=CARTESIAN_POINT ( 'NONE',  ( -1.630004931178638428, -7.334531690290998718, -435.2814510150427054 ) ) ;
#2656=ORIENTED_EDGE ( 'NONE', *, *, #4640, .F. ) ;
#2660=CARTESIAN_POINT ( 'NONE',  ( -14.74684780783305449, -5.500000000000000000, -439.3959507452315165 ) ) ;
#2682=( NAMED_UNIT ( * ) SI_UNIT ( $, .STERADIAN. ) SOLID_ANGLE_UNIT ( ) );
#2722=DIRECTION ( 'NONE',  ( 0.000000000000000000, 1.000000000000000000, 0.000000000000000000 ) ) ;
#2725=CARTESIAN_POINT ( 'NONE',  ( 7.995233561666595712, -7.656480000000000175, -523.7425978728656446 ) ) ;
#2729=EDGE_CURVE ( 'NONE', #5743, #4172, #6115, .T. ) ;
#2730=CARTESIAN_POINT ( 'NONE',  ( -1.867120547373915418, -7.452566320787000542, -434.7177009740820495 ) ) ;
#2737=EDGE_LOOP ( 'NONE', ( #9055, #9053, #1639, #5609, #7501 ) ) ;
#2742=CARTESIAN_POINT ( 'NONE',  ( -1.119552414421413511, -2.606163259540000610, -435.7158780125686235 ) ) ;
#2745=AXIS2_PLACEMENT_3D ( 'NONE', #2601, #7695, #3405 ) ;
#2752=CARTESIAN_POINT ( 'NONE',  ( 6.685859146470366277, -4.450907801408272135, -525.2546656924790796 ) ) ;
#2753=CARTESIAN_POINT ( 'NONE',  ( 7.584651611965206541, -5.651391369166294254, -525.7002755026068144 ) ) ;
#2755=ORIENTED_EDGE ( 'NONE', *, *, #8377, .T. ) ;
#2765=DIRECTION ( 'NONE',  ( -0.9712267471052594692, 0.000000000000000000, -0.2381566831044984178 ) ) ;
#2771=DIRECTION ( 'NONE',  ( -0.9712267471052612455, 0.000000000000000000, -0.2381566831044910626 ) ) ;
#2779=CARTESIAN_POINT ( 'NONE',  ( -0.5013770514288425906, -7.487604982435999368, -434.1602016854106978 ) ) ;
#2780=SHAPE_REPRESENTATION_RELATIONSHIP ( 'NONE' , 'NONE' ,  #4085, #5834 ) ;
#2798=CARTESIAN_POINT ( 'NONE',  ( 3.875825478601963248, -7.500000000000000000, -431.3627451401119970 ) ) ;
#2799=ADVANCED_FACE ( 'NONE', ( #6064 ), #7094, .F. ) ;
#2805=CARTESIAN_POINT ( 'NONE',  ( -12.86189863199293093, -5.758762107780500017, -438.9337381413729418 ) ) ;
#2806=CARTESIAN_POINT ( 'NONE',  ( -1.214899924133375331, -7.403467476614999043, -435.1227120718077686 ) ) ;
#2817=AXIS2_PLACEMENT_3D ( 'NONE', #8634, #3966, #3161 ) ;
#2837=AXIS2_PLACEMENT_3D ( 'NONE', #8842, #5662, #10447 ) ;
#2838=CARTESIAN_POINT ( 'NONE',  ( -1.207139762621110890, -7.484635725423999908, -434.4480596911860175 ) ) ;
#2844=CARTESIAN_POINT ( 'NONE',  ( -0.7342372444761647854, -7.494317894969175775, -434.2532513144291215 ) ) ;
#2856=CARTESIAN_POINT ( 'NONE',  ( 3.875825478601963248, -7.656480000000000175, -431.3627451401119970 ) ) ;
#2892=CARTESIAN_POINT ( 'NONE',  ( -0.6592970117152722187, -7.499999799589161853, -434.1413533491637509 ) ) ;
#2902=CARTESIAN_POINT ( 'NONE',  ( -2.301302514452984394, -7.114149834682999440, -436.1192177104634879 ) ) ;
#2925=VERTEX_POINT ( 'NONE', #10248 ) ;
#2930=ORIENTED_EDGE ( 'NONE', *, *, #407, .F. ) ;
#2943=DIRECTION ( 'NONE',  ( 0.000000000000000000, -1.000000000000000000, 0.000000000000000000 ) ) ;
#2950=CARTESIAN_POINT ( 'NONE',  ( -3.766936453924772277, -2.974863205562146007, -436.1437120911318743 ) ) ;
#2952=CARTESIAN_POINT ( 'NONE',  ( -1.999999999997229772, -2.500000000000000000, -409.4999999999571969 ) ) ;
#2957=LINE ( 'NONE', #6997, #6598 ) ;
#2961=FACE_OUTER_BOUND ( 'NONE', #7228, .T. ) ;
#2968=CARTESIAN_POINT ( 'NONE',  ( -0.8331085234012651775, -2.500134501855002078, -434.2559579827629364 ) ) ;
#2983=DIRECTION ( 'NONE',  ( -0.1124491875265152124, 0.000000000000000000, 0.9936574763089273121 ) ) ;
#2986=CARTESIAN_POINT ( 'NONE',  ( -0.6600535743662629962, -7.458390606629000885, -434.6313374073768614 ) ) ;
#2995=CARTESIAN_POINT ( 'NONE',  ( -1.333798302234134647, -7.456821208003824530, -434.5634752832991694 ) ) ;
#2999=CARTESIAN_POINT ( 'NONE',  ( -1.999999999997229772, -7.500000000000000000, -409.4999999999571969 ) ) ;
#3005=CARTESIAN_POINT ( 'NONE',  ( -11.69802267049820976, -4.081445891925754133, -438.6483114700716897 ) ) ;
#3007=CARTESIAN_POINT ( 'NONE',  ( -12.67039042656561243, -5.789333632204900937, -439.0231271474323762 ) ) ;
#3011=CARTESIAN_POINT ( 'NONE',  ( 6.353028986609323248, -4.484463380032637225, -524.9540790665465693 ) ) ;
#3013=ADVANCED_FACE ( 'NONE', ( #3690 ), #5514, .F. ) ;
#3020=CARTESIAN_POINT ( 'NONE',  ( -0.8897543176725906111, -2.502046059794002186, -434.2898615358246843 ) ) ;
#3024=FACE_OUTER_BOUND ( 'NONE', #5286, .T. ) ;
#3028=AXIS2_PLACEMENT_3D ( 'NONE', #2856, #8539, #5971 ) ;
#3040=ORIENTED_EDGE ( 'NONE', *, *, #9427, .F. ) ;
#3049=EDGE_CURVE ( 'NONE', #4096, #4227, #1159, .T. ) ;
#3063=EDGE_CURVE ( 'NONE', #9535, #4497, #8204, .T. ) ;
#3065=DIRECTION ( 'NONE',  ( -0.2381566831044910626, 0.000000000000000000, 0.9712267471052612455 ) ) ;
#3071=CARTESIAN_POINT ( 'NONE',  ( -14.83733877544362478, -5.575412435490171070, -439.0269195386780439 ) ) ;
#3072=CARTESIAN_POINT ( 'NONE',  ( -1.729952635784063331, -2.694803404275001313, -435.0907047969546966 ) ) ;
#3075=DIRECTION ( 'NONE',  ( -0.2381566831044917565, 0.000000000000000000, 0.9712267471052610235 ) ) ;
#3080=ORIENTED_EDGE ( 'NONE', *, *, #3319, .F. ) ;
#3107=CARTESIAN_POINT ( 'NONE',  ( 19.38368284813939013, -7.500000000000000000, -515.5999187775453265 ) ) ;
#3111=CARTESIAN_POINT ( 'NONE',  ( 28.53863984632670636, -2.500000000000000000, -506.8274460463252353 ) ) ;
#3126=CARTESIAN_POINT ( 'NONE',  ( -0.7288599747256179207, -2.498024261830999571, -434.1773087478343314 ) ) ;
#3133=EDGE_CURVE ( 'NONE', #10390, #9641, #5424, .T. ) ;
#3139=ORIENTED_EDGE ( 'NONE', *, *, #309, .T. ) ;
#3147=LINE ( 'NONE', #733, #9358 ) ;
#3149=EDGE_CURVE ( 'NONE', #574, #722, #1045, .T. ) ;
#3159=COLOUR_RGB ( '', 0.66274510, 0.83137255, 0.94901961) ;
#3161=DIRECTION ( 'NONE',  ( 1.000000000000000000, 0.000000000000000000, 0.000000000000000000 ) ) ;
#3165=LINE ( 'NONE', #3107, #6217 ) ;
#3184=CARTESIAN_POINT ( 'NONE',  ( -0.7166823250270980550, -2.498181146152001819, -434.1608823843793061 ) ) ;
#3188=STYLED_ITEM ( 'NONE', ( #7767 ), #5834 ) ;
#3191=CARTESIAN_POINT ( 'NONE',  ( -0.2949131312215419465, -7.545445293999001990, -434.0704074631209437 ) ) ;
#3195=CARTESIAN_POINT ( 'NONE',  ( -0.5535498271043974849, -7.499999952522999891, -434.2938920418101816 ) ) ;
#3203=DIRECTION ( 'NONE',  ( -0.000000000000000000, 1.000000000000000000, 0.000000000000000000 ) ) ;
#3216=EDGE_CURVE ( 'NONE', #146, #2925, #1238, .T. ) ;
#3222=CARTESIAN_POINT ( 'NONE',  ( -14.81438263496213814, -4.470068862813207922, -439.1205369730296297 ) ) ;
#3233=CARTESIAN_POINT ( 'NONE',  ( -3.707567269721498526, -7.033586184390685503, -436.1197384410193081 ) ) ;
#3236=CARTESIAN_POINT ( 'NONE',  ( -0.9356534891085935834, -2.545231261524000033, -435.0024077940244638 ) ) ;
#3237=CARTESIAN_POINT ( 'NONE',  ( -14.37110465573396212, -2.500000000000000000, -348.9812360766022721 ) ) ;
#3240=ADVANCED_FACE ( 'NONE', ( #2961 ), #6950, .F. ) ;
#3242=CARTESIAN_POINT ( 'NONE',  ( -1.837856579518353906, -7.344572662436001487, -434.9059567300546973 ) ) ;
#3277=CARTESIAN_POINT ( 'NONE',  ( -15.54870946350325767, -2.500000000000000000, -436.1258788022018393 ) ) ;
#3282=CARTESIAN_POINT ( 'NONE',  ( -5.399293614865643853, -7.500000000000000000, -410.3335483908228980 ) ) ;
#3283=CARTESIAN_POINT ( 'NONE',  ( -8.369756866907680504, -6.378185918057877934, -437.7466453813695466 ) ) ;
#3291=CARTESIAN_POINT ( 'NONE',  ( -0.7231407225213108969, -7.447240517548999961, -434.6679473676751400 ) ) ;
#3293=CARTESIAN_POINT ( 'NONE',  ( -16.17578790646000186, -2.500000000000000000, -433.5685902625999688 ) ) ;
#3295=ORIENTED_EDGE ( 'NONE', *, *, #8906, .F. ) ;
#3319=EDGE_CURVE ( 'NONE', #7492, #8716, #5526, .T. ) ;
#3334=CARTESIAN_POINT ( 'NONE',  ( -9.899579175599695802, -4.014440445723298723, -437.8439261505764648 ) ) ;
#3336=VECTOR ( 'NONE', #6671, 1000.000000000000000 ) ;
#3348=CIRCLE ( 'NONE', #5540, 3.500000000000005773 ) ;
#3350=CIRCLE ( 'NONE', #2837, 19.99999999999999289 ) ;
#3353=CARTESIAN_POINT ( 'NONE',  ( -0.3768446329310572995, -7.516309540199999084, -434.3911927895006784 ) ) ;
#3366=CARTESIAN_POINT ( 'NONE',  ( -4.143458015209706247, -7.288605749207033746, -435.5329359125040583 ) ) ;
#3369=CARTESIAN_POINT ( 'NONE',  ( -0.6468861588581515942, -7.500000251058999368, -434.1463208427667269 ) ) ;
#3390=CARTESIAN_POINT ( 'NONE',  ( -3.695312159471046076, -2.618857474173998057, -436.9735000885333989 ) ) ;
#3396=CARTESIAN_POINT ( 'NONE',  ( -1.762031438543397055, -7.488850308864000382, -434.6217938733590813 ) ) ;
#3404=CARTESIAN_POINT ( 'NONE',  ( 7.462474768419414595, -5.636463904742665676, -525.6703580967167682 ) ) ;
#3405=DIRECTION ( 'NONE',  ( 0.1283568000945425058, -0.9912279005316182445, 0.03149255590087908507 ) ) ;
#3419=CARTESIAN_POINT ( 'NONE',  ( -0.5695610819088786636, -7.500000013076999927, -434.2411922114832805 ) ) ;
#3441=CARTESIAN_POINT ( 'NONE',  ( -5.518773171133347866, -3.002193056125999515, -437.5009914653419401 ) ) ;
#3444=CARTESIAN_POINT ( 'NONE',  ( -1.873948611767810357, -7.500000000000000000, -349.2478646809746579 ) ) ;
#3447=CARTESIAN_POINT ( 'NONE',  ( -0.8444067271132583707, -2.512810845887640809, -434.3277856070802727 ) ) ;
#3448=FILL_AREA_STYLE ('',( #5208 ) ) ;
#3449=CARTESIAN_POINT ( 'NONE',  ( -11.92649270223300206, -6.242805967437002224, -437.6501176045007924 ) ) ;
#3454=DIRECTION ( 'NONE',  ( -0.9712267471052612455, 0.000000000000000000, -0.2381566831044910626 ) ) ;
#3456=CARTESIAN_POINT ( 'NONE',  ( 7.068287171791554080, -5.589036098012454268, -525.5562187735022235 ) ) ;
#3459=EDGE_CURVE ( 'NONE', #2618, #5593, #7886, .T. ) ;
#3469=VECTOR ( 'NONE', #9791, 1000.000000000000114 ) ;
#3486=SURFACE_STYLE_FILL_AREA ( #4292 ) ;
#3497=CARTESIAN_POINT ( 'NONE',  ( -1.399570435356993769, -2.031614869683998847, -436.0946480090682940 ) ) ;
#3500=FACE_OUTER_BOUND ( 'NONE', #10528, .T. ) ;
#3501=ORIENTED_EDGE ( 'NONE', *, *, #2260, .F. ) ;
#3504=CARTESIAN_POINT ( 'NONE',  ( -1.437790087008336881, -7.307863115514998675, -435.8454831066800921 ) ) ;
#3510=PLANE ( 'NONE',  #6133 ) ;
#3511=CARTESIAN_POINT ( 'NONE',  ( -1.999999999997229772, -2.500000000000000000, -409.4999999999571969 ) ) ;
#3519=EDGE_LOOP ( 'NONE', ( #7980, #7700, #4109, #4658 ) ) ;
#3521=AXIS2_PLACEMENT_3D ( 'NONE', #8895, #1644, #9916 ) ;
#3552=DIRECTION ( 'NONE',  ( -0.000000000000000000, 1.000000000000000000, 0.000000000000000000 ) ) ;
#3561=CARTESIAN_POINT ( 'NONE',  ( 8.920203998736104367, -5.829398780986294604, -525.5186553700950753 ) ) ;
#3576=LINE ( 'NONE', #7068, #7433 ) ;
#3594=ORIENTED_EDGE ( 'NONE', *, *, #1338, .F. ) ;
#3605=CARTESIAN_POINT ( 'NONE',  ( -0.5534908175310586653, -2.500000333914000006, -434.2941325283891274 ) ) ;
#3608=CARTESIAN_POINT ( 'NONE',  ( 19.38368284813939013, -2.500000000000000000, -515.5999187775453265 ) ) ;
#3612=CARTESIAN_POINT ( 'NONE',  ( 8.669822292802292552, -4.205922955401560692, -525.6304339756592299 ) ) ;
#3613=CARTESIAN_POINT ( 'NONE',  ( 7.445183927592051276, -5.634377803598318302, -525.6654729546380622 ) ) ;
#3633=CYLINDRICAL_SURFACE ( 'NONE', #6556, 2.000000000000033307 ) ;
#3634=VERTEX_POINT ( 'NONE', #1005 ) ;
#3644=ORIENTED_EDGE ( 'NONE', *, *, #4033, .T. ) ;
#3646=CARTESIAN_POINT ( 'NONE',  ( -0.6590269763235730993, -7.499720857620891579, -434.1629514920128372 ) ) ;
#3651=CARTESIAN_POINT ( 'NONE',  ( -14.37110465573396212, -2.500000000000000000, -348.9812360766022721 ) ) ;
#3653=CARTESIAN_POINT ( 'NONE',  ( -9.749126195418856611, -6.234330207147000813, -438.4907298204056474 ) ) ;
#3660=DIRECTION ( 'NONE',  ( -0.000000000000000000, 1.000000000000000000, 0.000000000000000000 ) ) ;
#3682=ORIENTED_EDGE ( 'NONE', *, *, #3149, .T. ) ;
#3690=FACE_OUTER_BOUND ( 'NONE', #7450, .T. ) ;
#3697=ORIENTED_EDGE ( 'NONE', *, *, #3049, .F. ) ;
#3698=CARTESIAN_POINT ( 'NONE',  ( -0.7938766977148212778, -7.490427039502949746, -434.2959395039480341 ) ) ;
#3715=CARTESIAN_POINT ( 'NONE',  ( 6.668310453960305750, -4.452685652811780415, -525.2390882416690374 ) ) ;
#3726=PRODUCT ( 'Upper Cutting Blade', 'Upper Cutting Blade', '', ( #9676 ) ) ;
#3729=ORIENTED_EDGE ( 'NONE', *, *, #5744, .F. ) ;
#3736=LINE ( 'NONE', #7024, #5911 ) ;
#3737=AXIS2_PLACEMENT_3D ( 'NONE', #752, #2, #805 ) ;
#3738=CARTESIAN_POINT ( 'NONE',  ( -0.7261718205266309845, -7.501926320342999333, -434.1735064888349029 ) ) ;
#3759=CARTESIAN_POINT ( 'NONE',  ( 6.666144892128035515, -4.452904620723932005, -525.2371525738265063 ) ) ;
#3769=CARTESIAN_POINT ( 'NONE',  ( -1.685183431873553461, -2.689364145315999099, -435.0748299022583296 ) ) ;
#3793=CARTESIAN_POINT ( 'NONE',  ( -1.367705781936138676, -7.477163225200000873, -434.5183335501718602 ) ) ;
#3810=CARTESIAN_POINT ( 'NONE',  ( -3.925578656483873274, -2.997421157293520544, -436.2071454890248674 ) ) ;
#3812=CARTESIAN_POINT ( 'NONE',  ( -1.399732096967147621, -7.968300772759999262, -436.0948124694132844 ) ) ;
#3830=FACE_OUTER_BOUND ( 'NONE', #7171, .T. ) ;
#3862=AXIS2_PLACEMENT_3D ( 'NONE', #6477, #9758, #5663 ) ;
#3869=CARTESIAN_POINT ( 'NONE',  ( -14.93448127581804385, -4.114638024020168316, -438.6307627169820194 ) ) ;
#3872=CARTESIAN_POINT ( 'NONE',  ( -0.5534908175310586653, -2.500000333914000006, -434.2941325283891274 ) ) ;
#3884=CARTESIAN_POINT ( 'NONE',  ( -1.793484850425402621, -2.651676682486001191, -434.8900474484831875 ) ) ;
#3912=EDGE_CURVE ( 'NONE', #574, #9045, #2345, .T. ) ;
#3913=ORIENTED_EDGE ( 'NONE', *, *, #5468, .T. ) ;
#3921=CARTESIAN_POINT ( 'NONE',  ( -14.95096017393944976, -4.021413106997576037, -438.5635601240937262 ) ) ;
#3936=CARTESIAN_POINT ( 'NONE',  ( -0.9394808717797451525, -2.588107745667998838, -434.7776290900898175 ) ) ;
#3960=ORIENTED_EDGE ( 'NONE', *, *, #138, .F. ) ;
#3966=DIRECTION ( 'NONE',  ( 0.000000000000000000, 0.000000000000000000, 1.000000000000000000 ) ) ;
#3977=DIRECTION ( 'NONE',  ( 0.2381566831044827082, 0.000000000000000000, -0.9712267471052632439 ) ) ;
#3985=EDGE_CURVE ( 'NONE', #4227, #6366, #3576, .T. ) ;
#3987=CARTESIAN_POINT ( 'NONE',  ( -1.588630714176977321, -2.677470159135998617, -435.0401446854098708 ) ) ;
#3992=CARTESIAN_POINT ( 'NONE',  ( -0.9146125851449583566, -7.458905582773998511, -434.9923621525751400 ) ) ;
#3995=FACE_BOUND ( 'NONE', #1870, .T. ) ;
#4008=DIRECTION ( 'NONE',  ( 0.7172627762233165782, -0.1147078669353000374, 0.6872963080852203532 ) ) ;
#4014=CARTESIAN_POINT ( 'NONE',  ( -2.737737974997910051, -2.627294679320482995, -435.0800218237813510 ) ) ;
#4027=CARTESIAN_POINT ( 'NONE',  ( -14.91834191543264154, -4.191152579685455848, -438.6965806410613027 ) ) ;
#4033=EDGE_CURVE ( 'NONE', #10001, #4938, #9478, .T. ) ;
#4043=CARTESIAN_POINT ( 'NONE',  ( -6.123887805759949288, -6.692614082003444764, -437.0035920074212186 ) ) ;
#4045=CARTESIAN_POINT ( 'NONE',  ( -14.95752314510466086, -6.038563360535726510, -438.5367956719984477 ) ) ;
#4046=CARTESIAN_POINT ( 'NONE',  ( -1.339600748765887639, -2.618129512416002669, -435.1727200896621639 ) ) ;
#4049=CYLINDRICAL_SURFACE ( 'NONE', #4967, 0.9999999999999971134 ) ;
#4053=CARTESIAN_POINT ( 'NONE',  ( -1.157768362637200621, -7.405868988916000539, -434.6424742340107059 ) ) ;
#4054=PLANE ( 'NONE',  #9090 ) ;
#4081=CARTESIAN_POINT ( 'NONE',  ( -14.91670604979136883, -4.198290335482643520, -438.7032518645799541 ) ) ;
#4083=ORIENTED_EDGE ( 'NONE', *, *, #8906, .T. ) ;
#4085=SHAPE_REPRESENTATION ( 'Upper Cutting Blade', ( #2817 ), #7989 ) ;
#4093=CARTESIAN_POINT ( 'NONE',  ( -1.582650547086741799, -7.339339277715000165, -435.1382983596024019 ) ) ;
#4095=CARTESIAN_POINT ( 'NONE',  ( -0.09974927406761666115, -2.336362244183999959, -434.1289336018982112 ) ) ;
#4096=VERTEX_POINT ( 'NONE', #454 ) ;
#4101=CARTESIAN_POINT ( 'NONE',  ( -1.439479021682663618, -7.379377528465000502, -434.7575680031760044 ) ) ;
#4105=ORIENTED_EDGE ( 'NONE', *, *, #2596, .T. ) ;
#4109=ORIENTED_EDGE ( 'NONE', *, *, #3912, .T. ) ;
#4123=DIRECTION ( 'NONE',  ( 0.9712267471052594692, 0.000000000000000000, 0.2381566831044984456 ) ) ;
#4141=CARTESIAN_POINT ( 'NONE',  ( -2.301732014548799388, -2.885986615635997676, -436.1194574627488691 ) ) ;
#4143=CARTESIAN_POINT ( 'NONE',  ( -14.98500449093754483, -5.000000000000000000, -438.4247239981262396 ) ) ;
#4147=APPLICATION_CONTEXT ( 'automotive_design' ) ;
#4148=CARTESIAN_POINT ( 'NONE',  ( -5.884114491779969036, -6.726235514389329317, -436.9226096605755174 ) ) ;
#4155=CARTESIAN_POINT ( 'NONE',  ( -0.4121893489828823420, -7.508048508167998847, -434.4353525244472394 ) ) ;
#4157=CARTESIAN_POINT ( 'NONE',  ( 1.399293614871181202, -7.500000000000000000, -408.6664516090914390 ) ) ;
#4159=ORIENTED_EDGE ( 'NONE', *, *, #5744, .T. ) ;
#4167=CARTESIAN_POINT ( 'NONE',  ( -5.399293614865643853, -2.500000000000000000, -410.3335483908228980 ) ) ;
#4172=VERTEX_POINT ( 'NONE', #8772 ) ;
#4185=ADVANCED_FACE ( 'NONE', ( #1583 ), #5603, .T. ) ;
#4188=DIRECTION ( 'NONE',  ( -0.000000000000000000, 1.000000000000000000, 0.000000000000000000 ) ) ;
#4197=CARTESIAN_POINT ( 'NONE',  ( -5.632814578931469640, -3.468398185772000097, -436.9796822201103055 ) ) ;
#4200=AXIS2_PLACEMENT_3D ( 'NONE', #4427, #1803, #2765 ) ;
#4211=CARTESIAN_POINT ( 'NONE',  ( 7.487150678296747408, -5.639452090671036366, -525.6770824513915841 ) ) ;
#4214=ORIENTED_EDGE ( 'NONE', *, *, #10035, .T. ) ;
#4227=VERTEX_POINT ( 'NONE', #6168 ) ;
#4249=ADVANCED_FACE ( 'NONE', ( #2468 ), #6604, .F. ) ;
#4251=CARTESIAN_POINT ( 'NONE',  ( -10.22024696720772319, -2.952319301924000161, -437.2166397675933354 ) ) ;
#4258=CARTESIAN_POINT ( 'NONE',  ( -5.872896638795078061, -6.657718028558998746, -436.3255011814985096 ) ) ;
#4261=CARTESIAN_POINT ( 'NONE',  ( -0.1804022943502615328, -2.368673688186001769, -434.4369549119049339 ) ) ;
#4277=EDGE_CURVE ( 'NONE', #890, #10001, #3165, .T. ) ;
#4285=ORIENTED_EDGE ( 'NONE', *, *, #7731, .T. ) ;
#4292=FILL_AREA_STYLE ('',( #1212 ) ) ;
#4301=AXIS2_PLACEMENT_3D ( 'NONE', #4143, #117, #8429 ) ;
#4302=CARTESIAN_POINT ( 'NONE',  ( -2.575517268146169325, -3.018520364412999868, -435.4821344709343975 ) ) ;
#4309=CARTESIAN_POINT ( 'NONE',  ( -1.120069929747936399, -7.393642214682999203, -435.7161955804480726 ) ) ;
#4311=CYLINDRICAL_SURFACE ( 'NONE', #8417, 12.49999999999999822 ) ;
#4314=CARTESIAN_POINT ( 'NONE',  ( 8.329446316317595134, -4.252668635446108070, -525.7144557534204523 ) ) ;
#4319=EDGE_CURVE ( 'NONE', #6718, #1530, #1927, .T. ) ;
#4324=ORIENTED_EDGE ( 'NONE', *, *, #5348, .F. ) ;
#4326=ORIENTED_EDGE ( 'NONE', *, *, #8377, .F. ) ;
#4357=EDGE_LOOP ( 'NONE', ( #526, #4825, #1100, #6386 ) ) ;
#4358=CARTESIAN_POINT ( 'NONE',  ( -0.7348864362710936238, -2.505735680000606536, -434.2545334094357941 ) ) ;
#4370=CARTESIAN_POINT ( 'NONE',  ( 6.127436559474321420, -5.500000000000000000, -524.5233678721955357 ) ) ;
#4377=ORIENTED_EDGE ( 'NONE', *, *, #6623, .T. ) ;
#4396=CARTESIAN_POINT ( 'NONE',  ( -0.7192419855824011554, -7.501856097319999250, -434.1639282888053799 ) ) ;
#4401=ORIENTED_EDGE ( 'NONE', *, *, #2596, .F. ) ;
#4416=CARTESIAN_POINT ( 'NONE',  ( 9.378959784071181360, -5.899999999999999467, -525.1866552614185366 ) ) ;
#4418=CARTESIAN_POINT ( 'NONE',  ( -13.49021588649789649, -5.672514732883807476, -439.0878092209056263 ) ) ;
#4427=CARTESIAN_POINT ( 'NONE',  ( -1.873948611767810357, -2.500000000000000000, -349.2478646809746579 ) ) ;
#4434=EDGE_CURVE ( 'NONE', #4096, #5868, #10043, .T. ) ;
#4435=CARTESIAN_POINT ( 'NONE',  ( -1.999999999997229772, -7.500000000000000000, -409.4999999999571969 ) ) ;
#4436=EDGE_LOOP ( 'NONE', ( #4083, #10241, #3729, #10115 ) ) ;
#4442=CARTESIAN_POINT ( 'NONE',  ( -0.5256544489318767388, -7.481870571157999805, -434.2361367940509354 ) ) ;
#4448=ORIENTED_EDGE ( 'NONE', *, *, #880, .F. ) ;
#4459=CARTESIAN_POINT ( 'NONE',  ( -5.631041015997348076, -6.531867497364999053, -436.9792595002378448 ) ) ;
#4470=DIRECTION ( 'NONE',  ( -0.9712269923486630541, -1.447945891862955814E-12, -0.2381556829751701188 ) ) ;
#4478=CARTESIAN_POINT ( 'NONE',  ( 30.17732799123041332, -3.250000000000000444, -426.5781481706914633 ) ) ;
#4479=ADVANCED_FACE ( 'NONE', ( #4868 ), #1696, .T. ) ;
#4482=EDGE_LOOP ( 'NONE', ( #2393, #4448, #2755, #7916 ) ) ;
#4487=CARTESIAN_POINT ( 'NONE',  ( -0.6303109507422630653, -7.465267904704998791, -434.3566826232884637 ) ) ;
#4497=VERTEX_POINT ( 'NONE', #4167 ) ;
#4498=CARTESIAN_POINT ( 'NONE',  ( -0.7615446691253315858, -7.492522473116027371, -434.2738182435463727 ) ) ;
#4500=ORIENTED_EDGE ( 'NONE', *, *, #3063, .T. ) ;
#4514=CARTESIAN_POINT ( 'NONE',  ( -1.999999999997229772, -7.500000000000000000, -409.4999999999571969 ) ) ;
#4519=CIRCLE ( 'NONE', #8469, 3.500000000000005773 ) ;
#4521=CARTESIAN_POINT ( 'NONE',  ( -14.84341486352006534, -5.586576249955223616, -439.0021406444614058 ) ) ;
#4531=ORIENTED_EDGE ( 'NONE', *, *, #7731, .F. ) ;
#4543=CARTESIAN_POINT ( 'NONE',  ( -1.771702344376552940, -7.457381197138002626, -434.6812846817269929 ) ) ;
#4560=CARTESIAN_POINT ( 'NONE',  ( 6.052780067456072999, -5.500000000000000000, -524.2189112390747141 ) ) ;
#4565=CARTESIAN_POINT ( 'NONE',  ( -3.694242493244381365, -7.381371554898000120, -436.9731892404009272 ) ) ;
#4574=CARTESIAN_POINT ( 'NONE',  ( -1.736715403303641825, -7.364240132115527082, -434.8724123522787863 ) ) ;
#4580=CARTESIAN_POINT ( 'NONE',  ( -0.5093080192647669868, -2.510898790358998767, -434.0830817482614634 ) ) ;
#4587=DIRECTION ( 'NONE',  ( -0.2381566831044910626, 0.000000000000000000, 0.9712267471052612455 ) ) ;
#4588=VERTEX_POINT ( 'NONE', #5614 ) ;
#4598=AXIS2_PLACEMENT_3D ( 'NONE', #2999, #10358, #8578 ) ;
#4599=CARTESIAN_POINT ( 'NONE',  ( -0.7199992077389804068, -7.501816435716998299, -434.1488804783251112 ) ) ;
#4607=CARTESIAN_POINT ( 'NONE',  ( -0.6665706852018948858, -7.499053979551672633, -434.1811903110214530 ) ) ;
#4614=CARTESIAN_POINT ( 'NONE',  ( -12.86189865087530038, -4.241237746457299451, -438.9337381460082952 ) ) ;
#4624=VECTOR ( 'NONE', #8310, 1000.000000000000000 ) ;
#4633=CARTESIAN_POINT ( 'NONE',  ( -14.74684780783305449, -5.500000000000000000, -439.3959507452315165 ) ) ;
#4634=CARTESIAN_POINT ( 'NONE',  ( -0.3527150178319009566, -2.477951988898999147, -434.3594990470874109 ) ) ;
#4640=EDGE_CURVE ( 'NONE', #4096, #890, #3147, .T. ) ;
#4652=CARTESIAN_POINT ( 'NONE',  ( -0.6650832026107983408, -7.510081290281999777, -434.8654298613620881 ) ) ;
#4658=ORIENTED_EDGE ( 'NONE', *, *, #7591, .T. ) ;
#4663=CARTESIAN_POINT ( 'NONE',  ( -1.424683970611967609, -7.451261721857263431, -434.6013510996728542 ) ) ;
#4664=CARTESIAN_POINT ( 'NONE',  ( -14.98500449093754483, -3.491150269972000064, -438.4247239981262396 ) ) ;
#4673=CARTESIAN_POINT ( 'NONE',  ( -13.22841485905253833, -6.750000122098000155, -437.9939945094035920 ) ) ;
#4681=ADVANCED_FACE ( 'NONE', ( #2450 ), #5719, .F. ) ;
#4687=VECTOR ( 'NONE', #9382, 1000.000000000000114 ) ;
#4689=CARTESIAN_POINT ( 'NONE',  ( -0.7524131241348165355, -2.498180379936999262, -434.1989882261000275 ) ) ;
#4690=EDGE_LOOP ( 'NONE', ( #1088, #3080, #5335, #4500 ) ) ;
#4695=APPLICATION_CONTEXT ( 'automotive_design' ) ;
#4702=CARTESIAN_POINT ( 'NONE',  ( -1.873948611767810357, -7.500000000000000000, -349.2478646809746579 ) ) ;
#4715=ORIENTED_EDGE ( 'NONE', *, *, #4277, .F. ) ;
#4717=EDGE_CURVE ( 'NONE', #78, #2925, #81, .T. ) ;
#4718=DIRECTION ( 'NONE',  ( -0.02133028834981354205, 0.000000000000000000, -0.9997724835175820779 ) ) ;
#4722=DIRECTION ( 'NONE',  ( 0.9712267471052612455, 7.261373026582001794E-09, 0.2381566831044910626 ) ) ;
#4733=DIRECTION ( 'NONE',  ( 0.000000000000000000, -1.000000000000000000, 0.000000000000000000 ) ) ;
#4747=CARTESIAN_POINT ( 'NONE',  ( -1.202539123581771952, -2.515137068876000637, -434.4460766357661328 ) ) ;
#4754=CARTESIAN_POINT ( 'NONE',  ( -0.5579452940971934005, -2.500000333914000006, -434.2759667279211158 ) ) ;
#4760=ORIENTED_EDGE ( 'NONE', *, *, #9427, .T. ) ;
#4769=CARTESIAN_POINT ( 'NONE',  ( -13.22841524816015202, -3.249999927714000147, -437.9939944912570127 ) ) ;
#4784=CARTESIAN_POINT ( 'NONE',  ( -14.84890384377945338, -4.402723804142927300, -438.9797560345791680 ) ) ;
#4798=CARTESIAN_POINT ( 'NONE',  ( -1.177149113458909824, -2.596052473566999641, -434.6509312389400748 ) ) ;
#4799=VERTEX_POINT ( 'NONE', #8404 ) ;
#4802=AXIS2_PLACEMENT_3D ( 'NONE', #5116, #1139, #238 ) ;
#4825=ORIENTED_EDGE ( 'NONE', *, *, #5112, .F. ) ;
#4839=AXIS2_PLACEMENT_3D ( 'NONE', #2367, #4733, #6327 ) ;
#4847=CARTESIAN_POINT ( 'NONE',  ( -2.291122522771679382, -7.236295659725429985, -435.5124405936905987 ) ) ;
#4849=CARTESIAN_POINT ( 'NONE',  ( -14.98500449093754838, -6.362323852810936486, -438.4247239981263533 ) ) ;
#4851=CARTESIAN_POINT ( 'NONE',  ( -0.8204922433515965396, -2.522492683188001461, -434.9474946677987077 ) ) ;
#4857=CARTESIAN_POINT ( 'NONE',  ( -0.8115155145918805379, -7.442392689726998967, -434.4760555596726022 ) ) ;
#4865=ORIENTED_EDGE ( 'NONE', *, *, #309, .F. ) ;
#4868=FACE_OUTER_BOUND ( 'NONE', #4436, .T. ) ;
#4871=DIRECTION ( 'NONE',  ( -0.000000000000000000, 1.000000000000000000, 0.000000000000000000 ) ) ;
#4875=EDGE_LOOP ( 'NONE', ( #2241, #401, #1236 ) ) ;
#4907=CARTESIAN_POINT ( 'NONE',  ( -0.3216191152362427585, -7.544227617881000825, -433.9889066583573367 ) ) ;
#4918=CARTESIAN_POINT ( 'NONE',  ( -1.873948611767810357, -7.500000000000000000, -349.2478646809746579 ) ) ;
#4921=EDGE_CURVE ( 'NONE', #5915, #8113, #2581, .T. ) ;
#4938=VERTEX_POINT ( 'NONE', #4997 ) ;
#4949=CARTESIAN_POINT ( 'NONE',  ( -14.97800895934490484, -6.224293360900853500, -438.4532524748601645 ) ) ;
#4954=ORIENTED_EDGE ( 'NONE', *, *, #5793, .T. ) ;
#4956=EDGE_CURVE ( 'NONE', #9192, #6833, #6670, .T. ) ;
#4957=CARTESIAN_POINT ( 'NONE',  ( -0.2499204815635852339, -7.611303227785001013, -434.5371318843381232 ) ) ;
#4967=AXIS2_PLACEMENT_3D ( 'NONE', #1576, #9687, #3075 ) ;
#4997=CARTESIAN_POINT ( 'NONE',  ( 10.54676984209158519, -7.500000000000000000, -347.8422498368975084 ) ) ;
#4999=CARTESIAN_POINT ( 'NONE',  ( -14.98500449093754483, -3.250000000000000444, -438.4247239981262396 ) ) ;
#5002=EDGE_CURVE ( 'NONE', #6684, #5593, #1326, .T. ) ;
#5004=CARTESIAN_POINT ( 'NONE',  ( -0.4024097121659061527, -7.571118624678998543, -434.6905673336279392 ) ) ;
#5013=ORIENTED_EDGE ( 'NONE', *, *, #7529, .F. ) ;
#5021=EDGE_LOOP ( 'NONE', ( #7132, #8006, #202, #3913, #943 ) ) ;
#5034=EDGE_CURVE ( 'NONE', #9136, #6684, #312, .T. ) ;
#5045=CARTESIAN_POINT ( 'NONE',  ( -13.01159837870191005, -3.814965662285999759, -437.8678677476697203 ) ) ;
#5051=LINE ( 'NONE', #10057, #3336 ) ;
#5053=CARTESIAN_POINT ( 'NONE',  ( -1.723960331780384880, -7.088439706543997687, -435.2349491625015503 ) ) ;
#5059=CARTESIAN_POINT ( 'NONE',  ( 9.231872887142856143, -4.123522793542388598, -525.3275970258257530 ) ) ;
#5060=CARTESIAN_POINT ( 'NONE',  ( 6.750050984497039330, -5.555647561257786471, -525.3462156153834712 ) ) ;
#5100=CARTESIAN_POINT ( 'NONE',  ( -9.752548285928396510, -3.766234771432999562, -438.4914339879979366 ) ) ;
#5103=ORIENTED_EDGE ( 'NONE', *, *, #138, .T. ) ;
#5105=( LENGTH_UNIT ( ) NAMED_UNIT ( * ) SI_UNIT ( .MILLI., .METRE. ) );
#5106=CARTESIAN_POINT ( 'NONE',  ( -13.28926923829693152, -6.170678168660001184, -437.9230910759725930 ) ) ;
#5112=EDGE_CURVE ( 'NONE', #1530, #9641, #2364, .T. ) ;
#5113=CARTESIAN_POINT ( 'NONE',  ( 8.350293318704649081, -4.249850286232732088, -525.7107168166273823 ) ) ;
#5114=B_SPLINE_CURVE_WITH_KNOTS ( 'NONE', 3,
 ( #9683, #446, #9578, #10326 ),
 .UNSPECIFIED., .F., .F.,
 ( 4, 4 ),
 ( 0.000000000000000000, 1.000000000000000000 ),
 .UNSPECIFIED. ) ;
#5115=CARTESIAN_POINT ( 'NONE',  ( 7.450340645337907297, -5.634999222355125070, -525.6669455952093131 ) ) ;
#5116=CARTESIAN_POINT ( 'NONE',  ( -12.99025666465511009, -6.750000000004000356, -438.9652312646727523 ) ) ;
#5153=CARTESIAN_POINT ( 'NONE',  ( -2.240834826158499382, -2.262508910126998174, -436.4488545418295757 ) ) ;
#5157=ORIENTED_EDGE ( 'NONE', *, *, #7529, .T. ) ;
#5161=CARTESIAN_POINT ( 'NONE',  ( -4.263294926846636912, -7.373286713554001892, -435.4918557313383758 ) ) ;
#5166=CARTESIAN_POINT ( 'NONE',  ( -16.17578790646000186, -7.500000000000000000, -433.5685902625999688 ) ) ;
#5167=CARTESIAN_POINT ( 'NONE',  ( -1.108984404642836541, -7.422390432154000628, -435.0786752202253638 ) ) ;
#5194=CARTESIAN_POINT ( 'NONE',  ( -0.5105614201597979962, -7.485013515304997256, -434.2009872517302256 ) ) ;
#5204=CARTESIAN_POINT ( 'NONE',  ( -11.92907573672570720, -3.757347598437999370, -437.6506565322029019 ) ) ;
#5207=CARTESIAN_POINT ( 'NONE',  ( -6.492778508125761405, -3.359043026927307274, -437.1259979785785958 ) ) ;
#5208=FILL_AREA_STYLE_COLOUR ( '', #3159 ) ;
#5214=CARTESIAN_POINT ( 'NONE',  ( -1.742616259932011413, -2.630534087998720683, -434.8631598522362083 ) ) ;
#5219=DIRECTION ( 'NONE',  ( 0.9712267471052594692, 0.000000000000000000, 0.2381566831044984456 ) ) ;
#5251=VERTEX_POINT ( 'NONE', #10197 ) ;
#5260=CARTESIAN_POINT ( 'NONE',  ( -4.094888478148218880, -3.021466021405220914, -436.2739009261703131 ) ) ;
#5261=CARTESIAN_POINT ( 'NONE',  ( -11.73256627085759973, -5.797438927934700281, -438.1636576033711776 ) ) ;
#5267=CARTESIAN_POINT ( 'NONE',  ( 6.280112539859566745, -5.511129512251558893, -524.8290735491510759 ) ) ;
#5273=CARTESIAN_POINT ( 'NONE',  ( -14.98500449093754483, -3.491150269972000064, -438.4247239981262396 ) ) ;
#5275=ORIENTED_EDGE ( 'NONE', *, *, #5348, .T. ) ;
#5286=EDGE_LOOP ( 'NONE', ( #3040, #2558, #5103, #9435 ) ) ;
#5293=CARTESIAN_POINT ( 'NONE',  ( -0.5691292782512946680, -7.474371670585999716, -434.2981779884299272 ) ) ;
#5310=CARTESIAN_POINT ( 'NONE',  ( -10.01353696546765804, -3.849175066121115485, -438.2031691364160793 ) ) ;
#5312=DIRECTION ( 'NONE',  ( -0.9997724835175819669, 0.000000000000000000, 0.02133028834981342756 ) ) ;
#5334=VERTEX_POINT ( 'NONE', #9065 ) ;
#5335=ORIENTED_EDGE ( 'NONE', *, *, #1454, .T. ) ;
#5340=CARTESIAN_POINT ( 'NONE',  ( -1.136797867647343807, -7.487797410750999028, -434.4157425830155717 ) ) ;
#5348=EDGE_CURVE ( 'NONE', #6305, #9271, #5935, .T. ) ;
#5352=CARTESIAN_POINT ( 'NONE',  ( -0.6929407895232514436, -7.497116523641391694, -434.2160164714800317 ) ) ;
#5353=DIRECTION ( 'NONE',  ( 0.9712267471052612455, 0.000000000000000000, 0.2381566831044910626 ) ) ;
#5355=VECTOR ( 'NONE', #9404, 1000.000000000000000 ) ;
#5359=CARTESIAN_POINT ( 'NONE',  ( -3.800715135322751514, -2.979668659210926940, -436.1572919893235962 ) ) ;
#5361=CARTESIAN_POINT ( 'NONE',  ( -7.533731257138555293, -6.615200789007997351, -438.0078122065712023 ) ) ;
#5386=VECTOR ( 'NONE', #4718, 1000.000000000000114 ) ;
#5403=ORIENTED_EDGE ( 'NONE', *, *, #313, .T. ) ;
#5408=CARTESIAN_POINT ( 'NONE',  ( -15.54870946350325767, -2.500000000000000000, -436.1258788022018393 ) ) ;
#5412=PRODUCT_DEFINITION_FORMATION_WITH_SPECIFIED_SOURCE ( 'ANY', '', #3726, .NOT_KNOWN. ) ;
#5416=DIRECTION ( 'NONE',  ( -0.000000000000000000, 1.000000000000000000, 0.000000000000000000 ) ) ;
#5420=EDGE_CURVE ( 'NONE', #722, #2333, #6974, .T. ) ;
#5424=LINE ( 'NONE', #6288, #7853 ) ;
#5431=CARTESIAN_POINT ( 'NONE',  ( -1.292800292905149417, -2.607107930518998362, -434.6991840609383644 ) ) ;
#5438=DIRECTION ( 'NONE',  ( 0.6918631112021742524, 0.000000000000000000, -0.7220286942758217252 ) ) ;
#5449=CARTESIAN_POINT ( 'NONE',  ( -0.2087206657751867478, -7.623098013552001007, -434.4789349137562340 ) ) ;
#5453=EDGE_LOOP ( 'NONE', ( #5013, #6295, #3594, #2019 ) ) ;
#5458=CARTESIAN_POINT ( 'NONE',  ( -1.725270327277327764, -7.432960991927813232, -434.7202860689826025 ) ) ;
#5460=EDGE_CURVE ( 'NONE', #5868, #2618, #5698, .T. ) ;
#5468=EDGE_CURVE ( 'NONE', #4588, #9045, #64, .T. ) ;
#5469=EDGE_LOOP ( 'NONE', ( #583, #4865, #3295, #4954 ) ) ;
#5486=CARTESIAN_POINT ( 'NONE',  ( -1.412886213222854792, -2.524971379295001928, -434.5374950603134039 ) ) ;
#5498=VERTEX_POINT ( 'NONE', #8385 ) ;
#5514=( BOUNDED_SURFACE ( )  B_SPLINE_SURFACE ( 3, 3, ( 
 ( #7670, #409, #4599, #6921, #4396, #3738, #9441, #8520, #9489, #2076, #1163, #8467, #7872, #521, #1114, #6105, #10194, #5340, #2838, #2130, #3793, #10089, #9392, #464, #4543, #2730, #5998, #10299 ),
 ( #9292, #7720, #2027, #1977, #2779, #5194, #4442, #362, #5293, #8566, #4487, #7766, #8133, #10549, #4857, #6463, #922, #771, #8284, #4053, #7382, #7329, #4101, #1370, #16, #6571, #9906, #3242 ),
 ( #9745, #10348, #4907, #3191, #8232, #9541, #2385, #822, #3353, #4155, #7276, #8185, #6519, #5651, #2986, #3291, #9855, #7081, #5759, #5708, #1735, #2494, #869, #6261, #2181, #9048, #8936, #2543 ),
 ( #8994, #6629, #2438, #571, #1683, #71, #7432, #10599, #5449, #4957, #5808, #9102, #5004, #1580, #1633, #8727, #4652, #9801, #7925, #3992, #1790, #5167, #2806, #1030, #9152, #8496, #7642, #2652 ) ),
 .UNSPECIFIED., .F., .F., .T. ) 
 B_SPLINE_SURFACE_WITH_KNOTS ( ( 4, 4 ),
 ( 4, 1, 1, 1, 1, 1, 1, 1, 1, 1, 1, 1, 1, 1, 1, 1, 1, 1, 1, 1, 1, 1, 1, 1, 1, 4 ),
 ( 0.000000000000000000, 1.000000000000000000 ),
 ( 0.07767058905990999185, 0.08939152241064000914, 0.1081359403480000037, 0.1244563457409999935, 0.1388518310880000051, 0.1526992796679999820, 0.1668709527589999908, 0.1819108867230999904, 0.1983140371714000039, 0.2165053751373000046, 0.2367746643099999937, 0.2591785502784000328, 0.2836740072810999824, 0.3102501903660999649, 0.3389525715886999579, 0.3700542176499000413, 0.4038975325576000253, 0.4407462203071000340, 0.4805450085883000155, 0.5231138182776999823, 0.5682755275442999965, 0.6162057510130999338, 0.6675662233626999953, 0.7230529014809999877, 0.7833591819763000563, 0.8073089092479999174 ),
 .UNSPECIFIED. ) 
 GEOMETRIC_REPRESENTATION_ITEM ( )  RATIONAL_B_SPLINE_SURFACE ( (
 ( 1.026133035016000061, 1.026133035016000061, 1.026133035016000061, 1.026133035016000061, 1.026133035016000061, 1.026133035016000061, 1.026133035016000061, 1.026133035016000061, 1.026133035016000061, 1.026133035016000061, 1.026133035016000061, 1.026133035016000061, 1.026133035016000061, 1.026133035016000061, 1.026133035016000061, 1.026133035016000061, 1.026133035016000061, 1.026133035016000061, 1.026133035016000061, 1.026133035016000061, 1.026133035016000061, 1.026133035016000061, 1.026133035016000061, 1.026133035016000061, 1.026133035016000061, 1.026133035016000061, 1.026133035016000061, 1.026133035016000061),
 ( 0.9912889883279000225, 0.9912889883279000225, 0.9912889883279000225, 0.9912889883279000225, 0.9912889883279000225, 0.9912889883279000225, 0.9912889883279000225, 0.9912889883279000225, 0.9912889883279000225, 0.9912889883279000225, 0.9912889883279000225, 0.9912889883279000225, 0.9912889883279000225, 0.9912889883279000225, 0.9912889883279000225, 0.9912889883279000225, 0.9912889883279000225, 0.9912889883279000225, 0.9912889883279000225, 0.9912889883279000225, 0.9912889883279000225, 0.9912889883279000225, 0.9912889883279000225, 0.9912889883279000225, 0.9912889883279000225, 0.9912889883279000225, 0.9912889883279000225, 0.9912889883279000225),
 ( 0.9912889883279000225, 0.9912889883279000225, 0.9912889883279000225, 0.9912889883279000225, 0.9912889883279000225, 0.9912889883279000225, 0.9912889883279000225, 0.9912889883279000225, 0.9912889883279000225, 0.9912889883279000225, 0.9912889883279000225, 0.9912889883279000225, 0.9912889883279000225, 0.9912889883279000225, 0.9912889883279000225, 0.9912889883279000225, 0.9912889883279000225, 0.9912889883279000225, 0.9912889883279000225, 0.9912889883279000225, 0.9912889883279000225, 0.9912889883279000225, 0.9912889883279000225, 0.9912889883279000225, 0.9912889883279000225, 0.9912889883279000225, 0.9912889883279000225, 0.9912889883279000225),
 ( 1.026133035016000061, 1.026133035016000061, 1.026133035016000061, 1.026133035016000061, 1.026133035016000061, 1.026133035016000061, 1.026133035016000061, 1.026133035016000061, 1.026133035016000061, 1.026133035016000061, 1.026133035016000061, 1.026133035016000061, 1.026133035016000061, 1.026133035016000061, 1.026133035016000061, 1.026133035016000061, 1.026133035016000061, 1.026133035016000061, 1.026133035016000061, 1.026133035016000061, 1.026133035016000061, 1.026133035016000061, 1.026133035016000061, 1.026133035016000061, 1.026133035016000061, 1.026133035016000061, 1.026133035016000061, 1.026133035016000061) ) ) 
 REPRESENTATION_ITEM ( '' )  SURFACE ( )  );
#5522=CARTESIAN_POINT ( 'NONE',  ( -0.6597201369859407860, -2.500000714168999938, -434.1397697187372273 ) ) ;
#5526=CIRCLE ( 'NONE', #7088, 3.500000000000005773 ) ;
#5536=CARTESIAN_POINT ( 'NONE',  ( -1.940862085953413141, -2.551169835479998316, -434.7454087554588682 ) ) ;
#5540=AXIS2_PLACEMENT_3D ( 'NONE', #5880, #255, #4123 ) ;
#5565=ORIENTED_EDGE ( 'NONE', *, *, #1759, .F. ) ;
#5571=VECTOR ( 'NONE', #519, 1000.000000000000000 ) ;
#5572=ADVANCED_FACE ( 'NONE', ( #5967 ), #379, .F. ) ;
#5578=CARTESIAN_POINT ( 'NONE',  ( -14.92114876071706320, -4.178597097557942952, -438.6851340455692139 ) ) ;
#5583=CARTESIAN_POINT ( 'NONE',  ( -1.662076676062295366, -2.666448017039082963, -434.9964371756940409 ) ) ;
#5593=VERTEX_POINT ( 'NONE', #3872 ) ;
#5594=CARTESIAN_POINT ( 'NONE',  ( -0.7274534428815968568, -2.498120223866999279, -434.1441721281535138 ) ) ;
#5597=DIRECTION ( 'NONE',  ( -0.9997724835175820779, -0.000000000000000000, 0.02133028834981354205 ) ) ;
#5603=PLANE ( 'NONE',  #8976 ) ;
#5609=ORIENTED_EDGE ( 'NONE', *, *, #4921, .F. ) ;
#5614=CARTESIAN_POINT ( 'NONE',  ( -14.98500449093754483, -6.750000000000000000, -438.4247239981262396 ) ) ;
#5617=ORIENTED_EDGE ( 'NONE', *, *, #373, .T. ) ;
#5619=EDGE_CURVE ( 'NONE', #4497, #9535, #5861, .T. ) ;
#5630=CARTESIAN_POINT ( 'NONE',  ( -14.97631232489547948, -3.822155571840307964, -438.4601715196498048 ) ) ;
#5644=CARTESIAN_POINT ( 'NONE',  ( -0.5500890142533868543, -2.522638648632998137, -434.2773879517249611 ) ) ;
#5651=CARTESIAN_POINT ( 'NONE',  ( -0.6014669115574718949, -7.469188726525000988, -434.5943147061385616 ) ) ;
#5652=CARTESIAN_POINT ( 'NONE',  ( -16.11962419174959393, -7.500000000000000000, -430.9361393731155658 ) ) ;
#5662=DIRECTION ( 'NONE',  ( -0.000000000000000000, 1.000000000000000000, 0.000000000000000000 ) ) ;
#5663=DIRECTION ( 'NONE',  ( -0.9712267471052612455, 0.000000000000000000, -0.2381566831044910626 ) ) ;
#5665=AXIS2_PLACEMENT_3D ( 'NONE', #2087, #5353, #2943 ) ;
#5669=ORIENTED_EDGE ( 'NONE', *, *, #6063, .F. ) ;
#5677=EDGE_CURVE ( 'NONE', #7332, #8193, #2619, .T. ) ;
#5690=EDGE_LOOP ( 'NONE', ( #5877, #5617, #3960, #7645, #7120, #6414, #1754, #5157, #8139 ) ) ;
#5698=LINE ( 'NONE', #6250, #3469 ) ;
#5707=PLANE ( 'NONE',  #6478 ) ;
#5708=CARTESIAN_POINT ( 'NONE',  ( -1.030241670742024773, -7.398214992874999396, -434.8184645790310014 ) ) ;
#5710=CARTESIAN_POINT ( 'NONE',  ( -0.5928343448393519344, -2.500000206366000288, -434.1985965821343143 ) ) ;
#5718=CARTESIAN_POINT ( 'NONE',  ( -1.813125098999968543, -7.427867185880000278, -434.7536662776001322 ) ) ;
#5719=PLANE ( 'NONE',  #3862 ) ;
#5736=DIRECTION ( 'NONE',  ( -0.2381566831044910626, 0.000000000000000000, 0.9712267471052612455 ) ) ;
#5743=VERTEX_POINT ( 'NONE', #3277 ) ;
#5744=EDGE_CURVE ( 'NONE', #5251, #10001, #9615, .T. ) ;
#5745=EDGE_CURVE ( 'NONE', #8113, #4172, #6554, .T. ) ;
#5753=CARTESIAN_POINT ( 'NONE',  ( -14.90548258804913928, -5.754348600474655129, -438.7490222628617857 ) ) ;
#5759=CARTESIAN_POINT ( 'NONE',  ( -0.9445117102953933808, -7.411175710731001232, -434.7797131905516039 ) ) ;
#5779=DIRECTION ( 'NONE',  ( -0.000000000000000000, 1.000000000000000000, 0.000000000000000000 ) ) ;
#5793=EDGE_CURVE ( 'NONE', #8235, #9192, #9818, .T. ) ;
#5796=CARTESIAN_POINT ( 'NONE',  ( -6.058905833985400946, -2.720859597169000388, -436.0408773327500285 ) ) ;
#5804=CARTESIAN_POINT ( 'NONE',  ( -0.1979899810951909478, -2.341947051001003199, -433.8401545479024435 ) ) ;
#5807=CARTESIAN_POINT ( 'NONE',  ( 6.864438614955176376, -4.432289485863268652, -525.3966049790363968 ) ) ;
#5808=CARTESIAN_POINT ( 'NONE',  ( -0.2960734841582018384, -7.598655014342003078, -434.5913138198718570 ) ) ;
#5824=CARTESIAN_POINT ( 'NONE',  ( -3.672986306062375750, -7.316704338766061078, -435.3862664917431857 ) ) ;
#5834=ADVANCED_BREP_SHAPE_REPRESENTATION ( '', ( #8937, #2817 ), #7989 ) ;
#5846=CARTESIAN_POINT ( 'NONE',  ( -13.10769452645968691, -4.328281264598399680, -438.3867334686859749 ) ) ;
#5848=EDGE_CURVE ( 'NONE', #7332, #3634, #9779, .T. ) ;
#5850=ORIENTED_EDGE ( 'NONE', *, *, #2410, .T. ) ;
#5853=CARTESIAN_POINT ( 'NONE',  ( -12.01210725212448338, -6.943331886975998124, -437.6899295328262838 ) ) ;
#5860=CARTESIAN_POINT ( 'NONE',  ( 8.142442032185543965, -5.722112424457679758, -525.7457260455852293 ) ) ;
#5861=CIRCLE ( 'NONE', #8781, 3.500000000000006217 ) ;
#5868=VERTEX_POINT ( 'NONE', #9668 ) ;
#5877=ORIENTED_EDGE ( 'NONE', *, *, #2729, .F. ) ;
#5878=CARTESIAN_POINT ( 'NONE',  ( -0.6596894340221253206, -7.499999891561000886, -434.1397621899948263 ) ) ;
#5880=CARTESIAN_POINT ( 'NONE',  ( -1.873948611767810357, -2.500000000000000000, -349.2478646809746579 ) ) ;
#5881=ORIENTED_EDGE ( 'NONE', *, *, #5677, .T. ) ;
#5904=CARTESIAN_POINT ( 'NONE',  ( -10.10898320382307602, -3.650023814309998116, -437.2731589972925121 ) ) ;
#5911=VECTOR ( 'NONE', #2983, 1000.000000000000114 ) ;
#5915=VERTEX_POINT ( 'NONE', #9248 ) ;
#5920=CARTESIAN_POINT ( 'NONE',  ( 8.650620448811780605, -5.791189843283389926, -525.6331420297578916 ) ) ;
#5926=LINE ( 'NONE', #9421, #6946 ) ;
#5935=B_SPLINE_CURVE_WITH_KNOTS ( 'NONE', 3,
 ( #5878, #3369, #2559, #7502, #3419, #6697, #9975 ),
 .UNSPECIFIED., .F., .F.,
 ( 4, 1, 1, 1, 4 ),
 ( 0.000000000000000000, 0.2500000000000000000, 0.5000000000000000000, 0.7500000000000000000, 1.000000000000000000 ),
 .UNSPECIFIED. ) ;
#5954=CARTESIAN_POINT ( 'NONE',  ( 9.378959784071181360, -5.899999999999999467, -525.1866552614185366 ) ) ;
#5965=CARTESIAN_POINT ( 'NONE',  ( -1.379544352527027007, -2.545980799917907600, -434.5827932828950679 ) ) ;
#5967=FACE_OUTER_BOUND ( 'NONE', #3519, .T. ) ;
#5971=DIRECTION ( 'NONE',  ( -0.9712267471052614676, 0.000000000000000000, -0.2381566831044902022 ) ) ;
#5972=CARTESIAN_POINT ( 'NONE',  ( 8.500452883955736283, -4.229385977086412396, -525.6786231025552070 ) ) ;
#5998=CARTESIAN_POINT ( 'NONE',  ( -1.924873525447142519, -7.449631413182002504, -434.7394372756328949 ) ) ;
#6001=DIRECTION ( 'NONE',  ( 0.000000000000000000, -1.000000000000000000, 0.000000000000000000 ) ) ;
#6009=CARTESIAN_POINT ( 'NONE',  ( -7.536255787234116710, -3.385256688352999088, -438.0084054756555929 ) ) ;
#6014=CARTESIAN_POINT ( 'NONE',  ( -1.267742039733871229, -2.539130078730544415, -434.5353378591038904 ) ) ;
#6022=CARTESIAN_POINT ( 'NONE',  ( 6.675319431708749640, -4.451976413186169879, -525.2453362690079075 ) ) ;
#6025=UNCERTAINTY_MEASURE_WITH_UNIT (LENGTH_MEASURE( 1.000000000000000082E-05 ), #8367, 'distance_accuracy_value', 'NONE');
#6036=AXIS2_PLACEMENT_3D ( 'NONE', #2798, #9362, #5312 ) ;
#6063=EDGE_CURVE ( 'NONE', #4799, #4588, #1985, .T. ) ;
#6064=FACE_OUTER_BOUND ( 'NONE', #191, .T. ) ;
#6086=CARTESIAN_POINT ( 'NONE',  ( -15.54870946350325767, -7.500000000000000000, -436.1258788022018393 ) ) ;
#6094=CARTESIAN_POINT ( 'NONE',  ( 28.53863984632670636, -7.500000000000000000, -506.8274460463252353 ) ) ;
#6105=CARTESIAN_POINT ( 'NONE',  ( -1.015842471293257887, -7.493001980645002114, -434.3570987632741094 ) ) ;
#6110=ORIENTED_EDGE ( 'NONE', *, *, #3985, .F. ) ;
#6115=LINE ( 'NONE', #5408, #9917 ) ;
#6121=CARTESIAN_POINT ( 'NONE',  ( -13.10769442058508716, -5.671717519033600219, -438.3867234666666945 ) ) ;
#6125=ADVANCED_FACE ( 'NONE', ( #1917 ), #3633, .T. ) ;
#6128=CARTESIAN_POINT ( 'NONE',  ( -1.582650547086741799, -7.339339277715000165, -435.1382983596024019 ) ) ;
#6133=AXIS2_PLACEMENT_3D ( 'NONE', #5166, #1136, #3454 ) ;
#6148=EDGE_LOOP ( 'NONE', ( #8606, #2112, #1599, #1353, #2274, #8092, #8018 ) ) ;
#6160=CARTESIAN_POINT ( 'NONE',  ( -0.8314117387865108677, -7.488021948898482272, -434.3195962711836842 ) ) ;
#6161=CARTESIAN_POINT ( 'NONE',  ( -14.37110465573396212, -7.500000000000000000, -348.9812360766022721 ) ) ;
#6168=CARTESIAN_POINT ( 'NONE',  ( 6.052780067456072999, -5.500000000000000000, -524.2189112390747141 ) ) ;
#6173=DIRECTION ( 'NONE',  ( 0.9627070496199739980, 0.1321637200910051047, 0.2360675490272045873 ) ) ;
#6176=ADVANCED_FACE ( 'NONE', ( #1419 ), #8140, .F. ) ;
#6202=VECTOR ( 'NONE', #7201, 1000.000000000000000 ) ;
#6217=VECTOR ( 'NONE', #9723, 1000.000000000000114 ) ;
#6223=CARTESIAN_POINT ( 'NONE',  ( -2.807317995047950987, -2.838317565875291937, -435.7570541054141131 ) ) ;
#6224=CARTESIAN_POINT ( 'NONE',  ( -12.86189865087530038, -4.241237746457299451, -438.9337381460082952 ) ) ;
#6231=DIRECTION ( 'NONE',  ( 0.1283609399493171599, 0.9912279006826364425, 0.03147567320362416182 ) ) ;
#6239=CARTESIAN_POINT ( 'NONE',  ( -0.7241641665009055373, -2.498143066284999936, -434.1460077833778541 ) ) ;
#6246=CARTESIAN_POINT ( 'NONE',  ( 6.877779018054728688, -2.500000000000000000, -527.5833393823892266 ) ) ;
#6250=CARTESIAN_POINT ( 'NONE',  ( 9.378959784071181360, -4.100000000000000533, -525.1866552614185366 ) ) ;
#6261=CARTESIAN_POINT ( 'NONE',  ( -1.433262749849905537, -7.342401167152001307, -434.9822336619507723 ) ) ;
#6270=CARTESIAN_POINT ( 'NONE',  ( -1.627435584940745361, -7.438904789989194022, -434.6825096147837826 ) ) ;
#6271=CYLINDRICAL_SURFACE ( 'NONE', #5665, 0.7499999999999997780 ) ;
#6272=MECHANICAL_DESIGN_GEOMETRIC_PRESENTATION_REPRESENTATION('',(#3188),#9707);
#6280=CARTESIAN_POINT ( 'NONE',  ( -6.872637154772029078, -3.412160298610301012, -437.2496588370372592 ) ) ;
#6282=CARTESIAN_POINT ( 'NONE',  ( -5.517019332057546244, -6.998165768227002204, -437.5004988621744246 ) ) ;
#6285=CARTESIAN_POINT ( 'NONE',  ( -1.582652182125599660, -2.660653890702000091, -435.1382991101020821 ) ) ;
#6288=CARTESIAN_POINT ( 'NONE',  ( 6.052780067456072999, -4.500000000000000888, -524.2189112390747141 ) ) ;
#6294=CARTESIAN_POINT ( 'NONE',  ( -0.2842986807686446182, -2.455579271718999035, -434.1368229023160552 ) ) ;
#6295=ORIENTED_EDGE ( 'NONE', *, *, #5002, .F. ) ;
#6305=VERTEX_POINT ( 'NONE', #9001 ) ;
#6311=VERTEX_POINT ( 'NONE', #6636 ) ;
#6327=DIRECTION ( 'NONE',  ( 0.9936574763089276452, 0.000000000000000000, 0.1124491875265132140 ) ) ;
#6345=CARTESIAN_POINT ( 'NONE',  ( -14.84121504900874911, -5.582427545768324784, -439.0111117078143934 ) ) ;
#6346=CARTESIAN_POINT ( 'NONE',  ( -1.029674599165786741, -2.507553075840000645, -434.3642002394484507 ) ) ;
#6347=ORIENTED_EDGE ( 'NONE', *, *, #5848, .T. ) ;
#6350=PLANE ( 'NONE',  #10289 ) ;
#6352=CARTESIAN_POINT ( 'NONE',  ( -15.54870946350325767, -7.500000000000000000, -436.1258788022018393 ) ) ;
#6366=VERTEX_POINT ( 'NONE', #2660 ) ;
#6367=VECTOR ( 'NONE', #556, 1000.000000000000000 ) ;
#6372=CARTESIAN_POINT ( 'NONE',  ( -2.040568488410468895, -2.585414927994879264, -434.8398312044259342 ) ) ;
#6384=CARTESIAN_POINT ( 'NONE',  ( -14.74684780783305449, -4.500000000000000888, -439.3959507452315165 ) ) ;
#6386=ORIENTED_EDGE ( 'NONE', *, *, #7743, .F. ) ;
#6393=ORIENTED_EDGE ( 'NONE', *, *, #5619, .F. ) ;
#6394=FACE_OUTER_BOUND ( 'NONE', #4690, .T. ) ;
#6395=EDGE_CURVE ( 'NONE', #5334, #6718, #10119, .T. ) ;
#6404=CARTESIAN_POINT ( 'NONE',  ( -1.629498688047873012, -2.665385218676999290, -435.2813193451249276 ) ) ;
#6414=ORIENTED_EDGE ( 'NONE', *, *, #770, .F. ) ;
#6457=CARTESIAN_POINT ( 'NONE',  ( -0.7400187527104828966, -2.555745218413001840, -434.6777242318867707 ) ) ;
#6463=CARTESIAN_POINT ( 'NONE',  ( -0.8690672964077537088, -7.435852491287998411, -434.5070751523649051 ) ) ;
#6470=DIRECTION ( 'NONE',  ( -0.9712267471052594692, 0.000000000000000000, -0.2381566831044984178 ) ) ;
#6477=CARTESIAN_POINT ( 'NONE',  ( -14.98500449093754483, -5.000000000000000000, -438.4247239981262396 ) ) ;
#6478=AXIS2_PLACEMENT_3D ( 'NONE', #8132, #10598, #8992 ) ;
#6509=CARTESIAN_POINT ( 'NONE',  ( -10.53397875998246036, -6.078358996281851390, -438.3628436008879703 ) ) ;
#6511=CARTESIAN_POINT ( 'NONE',  ( -14.87077422265778814, -5.645617090914123004, -438.8905664445195498 ) ) ;
#6513=DIRECTION ( 'NONE',  ( -0.02133028834981354205, 0.000000000000000000, -0.9997724835175820779 ) ) ;
#6519=CARTESIAN_POINT ( 'NONE',  ( -0.5472160415415407986, -7.479630378048000239, -434.5564753827179061 ) ) ;
#6523=VECTOR ( 'NONE', #4871, 1000.000000000000000 ) ;
#6545=( BOUNDED_SURFACE ( )  B_SPLINE_SURFACE ( 3, 3, ( 
 ( #7627, #1936, #10100, #4251, #8379, #5796, #9996, #9893, #2528, #9084 ),
 ( #9137, #5045, #5204, #5904, #2637, #908, #1014, #4302, #1722, #8328 ),
 ( #5846, #10051, #965, #3334, #9941, #4197, #165, #4141, #1069, #2742 ),
 ( #7472, #1882, #115, #5100, #6009, #3441, #3390, #5153, #3497, #2582 ) ),
 .UNSPECIFIED., .F., .F., .T. ) 
 B_SPLINE_SURFACE_WITH_KNOTS ( ( 4, 4 ),
 ( 4, 1, 1, 1, 1, 1, 1, 4 ),
 ( 0.000000000000000000, 1.000000000000000000 ),
 ( 0.1266979755386999917, 0.1849192355442000057, 0.3537297013212000185, 0.5087760485612999872, 0.6503402179949999695, 0.7796319686220000156, 0.8963498434801999704, 0.9600029233005999973 ),
 .UNSPECIFIED. ) 
 GEOMETRIC_REPRESENTATION_ITEM ( )  RATIONAL_B_SPLINE_SURFACE ( (
 ( 1.237059165673999983, 1.237059165673999983, 1.237059165673999983, 1.237059165673999983, 1.237059165673999983, 1.237059165673999983, 1.237059165673999983, 1.237059165673999983, 1.237059165673999983, 1.237059165673999983),
 ( 0.9209802781085000278, 0.9209802781085000278, 0.9209802781085000278, 0.9209802781085000278, 0.9209802781085000278, 0.9209802781085000278, 0.9209802781085000278, 0.9209802781085000278, 0.9209802781085000278, 0.9209802781085000278),
 ( 0.9209802781085000278, 0.9209802781085000278, 0.9209802781085000278, 0.9209802781085000278, 0.9209802781085000278, 0.9209802781085000278, 0.9209802781085000278, 0.9209802781085000278, 0.9209802781085000278, 0.9209802781085000278),
 ( 1.237059165673999983, 1.237059165673999983, 1.237059165673999983, 1.237059165673999983, 1.237059165673999983, 1.237059165673999983, 1.237059165673999983, 1.237059165673999983, 1.237059165673999983, 1.237059165673999983) ) ) 
 REPRESENTATION_ITEM ( '' )  SURFACE ( )  );
#6554=LINE ( 'NONE', #5522, #8096 ) ;
#6556=AXIS2_PLACEMENT_3D ( 'NONE', #2725, #355, #2071 ) ;
#6571=CARTESIAN_POINT ( 'NONE',  ( -1.761891692708837498, -7.351020573128999480, -434.8786339386260806 ) ) ;
#6574=CARTESIAN_POINT ( 'NONE',  ( -0.6597201369859407860, -2.500000714168999938, -434.1397697187372273 ) ) ;
#6582=B_SPLINE_CURVE_WITH_KNOTS ( 'NONE', 3,
 ( #1898, #4418, #129, #10013 ),
 .UNSPECIFIED., .F., .F.,
 ( 4, 4 ),
 ( 0.000000000000000000, 1.000000000000000000 ),
 .UNSPECIFIED. ) ;
#6598=VECTOR ( 'NONE', #650, 1000.000000000000000 ) ;
#6604=PLANE ( 'NONE',  #10346 ) ;
#6609=AXIS2_PLACEMENT_3D ( 'NONE', #4435, #302, #400 ) ;
#6621=SURFACE_STYLE_USAGE ( .BOTH. , #1022 ) ;
#6623=EDGE_CURVE ( 'NONE', #8193, #6311, #2057, .T. ) ;
#6629=CARTESIAN_POINT ( 'NONE',  ( -0.1882039595137465215, -7.659278717692999727, -433.8551617668519498 ) ) ;
#6636=CARTESIAN_POINT ( 'NONE',  ( -15.16362200326591569, -7.500000000000000000, -437.6963039377973246 ) ) ;
#6637=ORIENTED_EDGE ( 'NONE', *, *, #373, .F. ) ;
#6643=CARTESIAN_POINT ( 'NONE',  ( -5.561812994916270014, -7.204029759630539154, -435.9619401370908918 ) ) ;
#6670=LINE ( 'NONE', #3651, #9518 ) ;
#6671=DIRECTION ( 'NONE',  ( 0.000000000000000000, -1.000000000000000000, 0.000000000000000000 ) ) ;
#6678=CARTESIAN_POINT ( 'NONE',  ( 8.494641066709883503, -5.769732973146090238, -525.6795250154979158 ) ) ;
#6680=ADVANCED_FACE ( 'NONE', ( #9684 ), #8814, .F. ) ;
#6684=VERTEX_POINT ( 'NONE', #9 ) ;
#6697=CARTESIAN_POINT ( 'NONE',  ( -0.5580839194863698172, -7.499999952522999891, -434.2754015600911544 ) ) ;
#6702=CARTESIAN_POINT ( 'NONE',  ( 19.38368284813939013, -7.500000000000000000, -515.5999187775453265 ) ) ;
#6718=VERTEX_POINT ( 'NONE', #4999 ) ;
#6726=SURFACE_STYLE_FILL_AREA ( #3448 ) ;
#6762=DIRECTION ( 'NONE',  ( -0.9712267471052594692, 0.000000000000000000, -0.2381566831044984178 ) ) ;
#6777=CARTESIAN_POINT ( 'NONE',  ( 19.38368284813939013, -2.500000000000000000, -515.5999187775453265 ) ) ;
#6780=DIRECTION ( 'NONE',  ( -0.9712267471052594692, 0.000000000000000000, -0.2381566831044984178 ) ) ;
#6818=SURFACE_SIDE_STYLE ('',( #3486 ) ) ;
#6826=EDGE_LOOP ( 'NONE', ( #7475, #10185, #6347, #6637 ) ) ;
#6833=VERTEX_POINT ( 'NONE', #6161 ) ;
#6836=ADVANCED_FACE ( 'NONE', ( #9450 ), #6271, .T. ) ;
#6857=ORIENTED_EDGE ( 'NONE', *, *, #7743, .T. ) ;
#6861=EDGE_CURVE ( 'NONE', #1530, #5334, #10307, .T. ) ;
#6879=ORIENTED_EDGE ( 'NONE', *, *, #1682, .T. ) ;
#6913=EDGE_LOOP ( 'NONE', ( #1121, #1390 ) ) ;
#6920=ADVANCED_FACE ( 'NONE', ( #8388 ), #4311, .T. ) ;
#6921=CARTESIAN_POINT ( 'NONE',  ( -0.7165654159986467597, -7.501783096816999397, -434.1553209429059166 ) ) ;
#6929=CARTESIAN_POINT ( 'NONE',  ( -0.7115441411924354753, -7.495838068657331377, -434.2340922344590695 ) ) ;
#6932=DIRECTION ( 'NONE',  ( 0.2381566831044910626, 0.000000000000000000, -0.9712267471052612455 ) ) ;
#6946=VECTOR ( 'NONE', #6956, 1000.000000000000114 ) ;
#6950=PLANE ( 'NONE',  #2628 ) ;
#6956=DIRECTION ( 'NONE',  ( 0.2381566830310488381, -5.671339926113999656E-10, -0.9712267471232701732 ) ) ;
#6974=B_SPLINE_CURVE_WITH_KNOTS ( 'NONE', 3,
 ( #4093, #9037, #4847, #2378, #2429, #8985, #759, #3233, #8177, #10538, #7070, #1309, #8122, #7371, #4148, #4043, #10337, #3283, #6509, #7320 ),
 .UNSPECIFIED., .F., .F.,
 ( 4, 1, 1, 1, 1, 1, 1, 2, 2, 1, 1, 2, 2, 4 ),
 ( 0.000000000000000000, 0.1250000000000086875, 0.1875000000000131006, 0.2187500000000181799, 0.2343750000000180134, 0.2421875000000205114, 0.2460937500000218159, 0.2480468750000249800, 0.2500000000000281442, 0.3750000000000131561, 0.4375000000000058287, 0.4687500000000042744, 0.5000000000000027756, 1.000000000000000000 ),
 .UNSPECIFIED. ) ;
#6989=CARTESIAN_POINT ( 'NONE',  ( -0.6597201369859407860, -2.500000714168999938, -434.1397697187372273 ) ) ;
#6997=CARTESIAN_POINT ( 'NONE',  ( 1.399293614871181202, -7.500000000000000000, -408.6664516090914390 ) ) ;
#7001=DIRECTION ( 'NONE',  ( 0.9712267471052594692, 0.000000000000000000, 0.2381566831044984456 ) ) ;
#7014=EDGE_CURVE ( 'NONE', #6311, #6305, #9894, .T. ) ;
#7024=CARTESIAN_POINT ( 'NONE',  ( 28.53863984632670636, -2.500000000000000000, -506.8274460463252353 ) ) ;
#7035=CARTESIAN_POINT ( 'NONE',  ( -0.9751833592927913186, -7.478962837042861800, -434.3989537440571667 ) ) ;
#7044=CARTESIAN_POINT ( 'NONE',  ( -5.178550450922173809, -3.174732006113173188, -436.6812520500867549 ) ) ;
#7046=CARTESIAN_POINT ( 'NONE',  ( -3.784291777249242816, -6.824938403275000454, -436.5423981522574763 ) ) ;
#7062=CARTESIAN_POINT ( 'NONE',  ( -1.050554280480674452, -2.604844966689999097, -434.8275985566710347 ) ) ;
#7068=CARTESIAN_POINT ( 'NONE',  ( 6.052780067456072999, -5.500000000000000000, -524.2189112390747141 ) ) ;
#7070=CARTESIAN_POINT ( 'NONE',  ( -3.753597148019404806, -7.027035274121325337, -436.1383244323657777 ) ) ;
#7079=VECTOR ( 'NONE', #10471, 1000.000000000000000 ) ;
#7081=CARTESIAN_POINT ( 'NONE',  ( -0.8648435279641549789, -7.423678894978000820, -434.7417815575237796 ) ) ;
#7088=AXIS2_PLACEMENT_3D ( 'NONE', #4514, #7794, #7001 ) ;
#7091=CARTESIAN_POINT ( 'NONE',  ( -0.6578543451058023184, -7.499974772742706186, -434.1490756834378431 ) ) ;
#7093=VECTOR ( 'NONE', #6001, 1000.000000000000000 ) ;
#7094=CYLINDRICAL_SURFACE ( 'NONE', #4598, 3.500000000000006217 ) ;
#7099=CARTESIAN_POINT ( 'NONE',  ( -12.95168232056959212, -5.749022766740000456, -439.0697820409906171 ) ) ;
#7110=CARTESIAN_POINT ( 'NONE',  ( -14.85829447703713235, -5.615530704401715312, -438.9414600939686011 ) ) ;
#7112=CARTESIAN_POINT ( 'NONE',  ( -0.6495235857412369196, -2.539793227551998545, -434.6255535651486639 ) ) ;
#7120=ORIENTED_EDGE ( 'NONE', *, *, #342, .F. ) ;
#7125=ORIENTED_EDGE ( 'NONE', *, *, #6623, .F. ) ;
#7132=ORIENTED_EDGE ( 'NONE', *, *, #10035, .F. ) ;
#7134=LINE ( 'NONE', #9654, #5386 ) ;
#7146=CARTESIAN_POINT ( 'NONE',  ( -14.88932286584991438, -4.303667523461871980, -438.8149232244517179 ) ) ;
#7160=CARTESIAN_POINT ( 'NONE',  ( -14.76420639513456301, -5.500000000000000000, -439.3251606919798178 ) ) ;
#7161=CARTESIAN_POINT ( 'NONE',  ( -1.111851599903384891, -2.511083096523998748, -434.4041198421772947 ) ) ;
#7162=ORIENTED_EDGE ( 'NONE', *, *, #5420, .T. ) ;
#7171=EDGE_LOOP ( 'NONE', ( #4105, #5565, #4531, #8461 ) ) ;
#7201=DIRECTION ( 'NONE',  ( -0.000000000000000000, 1.000000000000000000, 0.000000000000000000 ) ) ;
#7216=CARTESIAN_POINT ( 'NONE',  ( -0.3553996609399175943, -2.459433156087002192, -433.9334582789244905 ) ) ;
#7223=PRODUCT_DEFINITION_CONTEXT ( 'detailed design', #4695, 'design' ) ;
#7228=EDGE_LOOP ( 'NONE', ( #4285, #6110, #3697, #907, #1253, #6879, #7162 ) ) ;
#7252=CARTESIAN_POINT ( 'NONE',  ( -14.98500449093754838, -3.629407339799118226, -438.4247239981262965 ) ) ;
#7256=EDGE_CURVE ( 'NONE', #9641, #9136, #1760, .T. ) ;
#7269=CARTESIAN_POINT ( 'NONE',  ( -0.4853341206058132129, -2.507971610063000956, -434.5088091749634600 ) ) ;
#7276=CARTESIAN_POINT ( 'NONE',  ( -0.4523805927985417030, -7.499149346347998346, -434.4772701732684936 ) ) ;
#7306=CARTESIAN_POINT ( 'NONE',  ( -14.98500449093754483, -4.500000000000000888, -438.4247239981262396 ) ) ;
#7311=CARTESIAN_POINT ( 'NONE',  ( -16.11962419174959393, -7.500000000000000000, -430.9361393731155658 ) ) ;
#7312=ORIENTED_EDGE ( 'NONE', *, *, #1527, .T. ) ;
#7313=B_SPLINE_CURVE_WITH_KNOTS ( 'NONE', 3,
 ( #1842, #5059, #7486, #3612, #5972, #10110, #2541, #5113, #1029, #4314, #180, #2597, #234, #9263, #5807, #1896, #9100, #2752, #6022, #3715, #3759, #3011, #385, #1343 ),
 .UNSPECIFIED., .F., .F.,
 ( 4, 1, 1, 1, 1, 1, 2, 2, 2, 1, 1, 1, 1, 1, 2, 2, 4 ),
 ( 0.000000000000000000, 0.1250000000000436873, 0.1875000000000811018, 0.2187500000000887901, 0.2343750000000931477, 0.2421875000000953404, 0.2460937500000959233, 0.2500000000000964784, 0.4999999999999881206, 0.6249999999999342748, 0.6874999999999298339, 0.7187499999999547029, 0.7343749999999963363, 0.7421875000000170974, 0.7460937500000278666, 0.7500000000000385247, 1.000000000000000000 ),
 .UNSPECIFIED. ) ;
#7320=CARTESIAN_POINT ( 'NONE',  ( -12.86189863199293093, -5.758762107780500017, -438.9337381413729418 ) ) ;
#7323=CARTESIAN_POINT ( 'NONE',  ( -1.584100026069928724, -2.658208447551997811, -435.2648446327503962 ) ) ;
#7329=CARTESIAN_POINT ( 'NONE',  ( -1.339266931960580331, -7.388578682852002366, -434.7178764703356251 ) ) ;
#7330=DIRECTION ( 'NONE',  ( 0.000000000000000000, -1.000000000000000000, -0.000000000000000000 ) ) ;
#7332=VERTEX_POINT ( 'NONE', #5652 ) ;
#7371=CARTESIAN_POINT ( 'NONE',  ( -5.530027647682731917, -6.775927878003381366, -436.8017055862294455 ) ) ;
#7372=CARTESIAN_POINT ( 'NONE',  ( -14.93900900976164969, -5.907301249192538961, -438.6122981656100137 ) ) ;
#7373=CARTESIAN_POINT ( 'NONE',  ( -0.6109814867824735485, -2.478111245608000779, -434.8347466770483152 ) ) ;
#7377=CIRCLE ( 'NONE', #2745, 1.000009933063999545 ) ;
#7379=ORIENTED_EDGE ( 'NONE', *, *, #8075, .T. ) ;
#7382=CARTESIAN_POINT ( 'NONE',  ( -1.245518217540318773, -7.397396954862998086, -434.6795757337810642 ) ) ;
#7399=CARTESIAN_POINT ( 'NONE',  ( 1.399293614871181202, -2.500000000000000000, -408.6664516090914390 ) ) ;
#7421=CARTESIAN_POINT ( 'NONE',  ( -1.638209378284813722, -2.561752193325623317, -434.6868264169996223 ) ) ;
#7432=CARTESIAN_POINT ( 'NONE',  ( -0.1421619115827766622, -7.644091901224001617, -434.3437170732802315 ) ) ;
#7433=VECTOR ( 'NONE', #4587, 1000.000000000000000 ) ;
#7437=ORIENTED_EDGE ( 'NONE', *, *, #3985, .T. ) ;
#7450=EDGE_LOOP ( 'NONE', ( #3682, #8862, #4324, #4214 ) ) ;
#7457=VECTOR ( 'NONE', #6513, 1000.000000000000114 ) ;
#7469=AXIS2_PLACEMENT_3D ( 'NONE', #2025, #7764, #7870 ) ;
#7472=CARTESIAN_POINT ( 'NONE',  ( -12.95168464415343834, -4.250977063078799745, -439.0697824306216717 ) ) ;
#7474=FACE_OUTER_BOUND ( 'NONE', #4875, .T. ) ;
#7475=ORIENTED_EDGE ( 'NONE', *, *, #1952, .F. ) ;
#7481=CARTESIAN_POINT ( 'NONE',  ( -0.4215672289900458392, -2.433748306090999236, -434.7071814881026057 ) ) ;
#7486=CARTESIAN_POINT ( 'NONE',  ( 8.989791091710285897, -4.160326409263540803, -525.4993780678859139 ) ) ;
#7492=VERTEX_POINT ( 'NONE', #4157 ) ;
#7498=ADVANCED_FACE ( 'NONE', ( #720, #3995, #10551 ), #4054, .F. ) ;
#7501=ORIENTED_EDGE ( 'NONE', *, *, #9391, .F. ) ;
#7502=CARTESIAN_POINT ( 'NONE',  ( -0.5933647373784489698, -7.500000025448000152, -434.1978076166600431 ) ) ;
#7503=CARTESIAN_POINT ( 'NONE',  ( -15.16362200326591569, -3.250000000000000444, -437.6963039377973246 ) ) ;
#7522=DIRECTION ( 'NONE',  ( -0.9627072963110285819, 0.1321637200909012433, -0.2360665429942227778 ) ) ;
#7528=CARTESIAN_POINT ( 'NONE',  ( -7.893353328029269811, -6.500255900689999145, -436.7904933931527580 ) ) ;
#7529=EDGE_CURVE ( 'NONE', #5593, #8113, #8495, .T. ) ;
#7567=CARTESIAN_POINT ( 'NONE',  ( -14.98500449093754483, -3.250000000000000444, -438.4247239981262396 ) ) ;
#7578=CARTESIAN_POINT ( 'NONE',  ( -1.813125407131493949, -2.572135581867000198, -434.7536649739391237 ) ) ;
#7582=CARTESIAN_POINT ( 'NONE',  ( -1.873948611767810357, -2.500000000000000000, -349.2478646809746579 ) ) ;
#7587=CARTESIAN_POINT ( 'NONE',  ( 7.750957818532088872, -5.672096822788666337, -525.7290262469028903 ) ) ;
#7591=EDGE_CURVE ( 'NONE', #9045, #2333, #1886, .T. ) ;
#7592=VECTOR ( 'NONE', #3660, 1000.000000000000000 ) ;
#7597=ORIENTED_EDGE ( 'NONE', *, *, #3133, .F. ) ;
#7627=CARTESIAN_POINT ( 'NONE',  ( -13.35722287852525270, -3.136587239007000871, -438.0342749280858925 ) ) ;
#7633=CIRCLE ( 'NONE', #7469, 12.50000000000000178 ) ;
#7635=CARTESIAN_POINT ( 'NONE',  ( -13.08165157527891331, -6.879863062859000955, -437.9641712690918780 ) ) ;
#7642=CARTESIAN_POINT ( 'NONE',  ( -1.612612246911211633, -7.337280841968000011, -435.2751398942043579 ) ) ;
#7645=ORIENTED_EDGE ( 'NONE', *, *, #5793, .F. ) ;
#7648=EDGE_LOOP ( 'NONE', ( #5669, #4401, #1365 ) ) ;
#7652=COLOUR_RGB ( '', 0.66274510, 0.83137255, 0.94901961) ;
#7663=ORIENTED_EDGE ( 'NONE', *, *, #5112, .T. ) ;
#7670=CARTESIAN_POINT ( 'NONE',  ( -0.7282841184975303861, -7.501884272294999434, -434.1436991062553261 ) ) ;
#7693=CARTESIAN_POINT ( 'NONE',  ( 7.974011974874644082, -5.700385244905218585, -525.7480461867619397 ) ) ;
#7695=DIRECTION ( 'NONE',  ( -0.9627071798692586890, -0.1321637200910267818, -0.2360670178569624911 ) ) ;
#7700=ORIENTED_EDGE ( 'NONE', *, *, #3149, .F. ) ;
#7715=ORIENTED_EDGE ( 'NONE', *, *, #9566, .T. ) ;
#7718=CARTESIAN_POINT ( 'NONE',  ( -5.399293614865643853, -7.500000000000000000, -410.3335483908228980 ) ) ;
#7720=CARTESIAN_POINT ( 'NONE',  ( -0.5335076011871895396, -7.487113625182997723, -434.0440531843738086 ) ) ;
#7731=EDGE_CURVE ( 'NONE', #2333, #6366, #6582, .T. ) ;
#7738=LINE ( 'NONE', #3608, #9265 ) ;
#7742=CARTESIAN_POINT ( 'NONE',  ( -0.4166032843586319201, -7.500000000000000000, -434.8523737515589573 ) ) ;
#7743=EDGE_CURVE ( 'NONE', #9136, #5334, #7377, .T. ) ;
#7764=DIRECTION ( 'NONE',  ( 0.000000000000000000, -1.000000000000000000, 0.000000000000000000 ) ) ;
#7766=CARTESIAN_POINT ( 'NONE',  ( -0.6682209595297889937, -7.460089650475999257, -434.3860247085133324 ) ) ;
#7767=PRESENTATION_STYLE_ASSIGNMENT (( #9293 ) ) ;
#7794=DIRECTION ( 'NONE',  ( -0.000000000000000000, 1.000000000000000000, 0.000000000000000000 ) ) ;
#7800=CARTESIAN_POINT ( 'NONE',  ( -13.22841710535096027, -3.249999999997000177, -437.9939891937848984 ) ) ;
#7814=EDGE_LOOP ( 'NONE', ( #7379, #3501, #1957, #2032 ) ) ;
#7817=LINE ( 'NONE', #7718, #5571 ) ;
#7836=CARTESIAN_POINT ( 'NONE',  ( -3.783028835520242161, -2.977152670199212370, -436.1501852806630950 ) ) ;
#7853=VECTOR ( 'NONE', #3065, 1000.000000000000000 ) ;
#7856=CARTESIAN_POINT ( 'NONE',  ( -0.7870641098475030795, -2.498849777199999789, -434.2253465126299261 ) ) ;
#7870=DIRECTION ( 'NONE',  ( 0.9936574763089276452, 0.000000000000000000, 0.1124491875265132140 ) ) ;
#7872=CARTESIAN_POINT ( 'NONE',  ( -0.8774468747956698511, -7.498360183982002880, -434.2824815778216703 ) ) ;
#7881=CARTESIAN_POINT ( 'NONE',  ( -0.8741371413883790575, -7.485309303923605384, -434.3446856359637991 ) ) ;
#7886=LINE ( 'NONE', #1332, #5355 ) ;
#7889=CARTESIAN_POINT ( 'NONE',  ( -7.253510651729878411, -3.465370319632318896, -437.3721018849337270 ) ) ;
#7891=CARTESIAN_POINT ( 'NONE',  ( -1.093860234711317325, -8.065417674857998875, -435.9303386687636248 ) ) ;
#7904=CARTESIAN_POINT ( 'NONE',  ( -14.78950287887041526, -5.511224176445043810, -439.2219991040214495 ) ) ;
#7905=CARTESIAN_POINT ( 'NONE',  ( -0.3057234697441956195, -2.465012315298997780, -434.2611651091350495 ) ) ;
#7916=ORIENTED_EDGE ( 'NONE', *, *, #4717, .T. ) ;
#7925=CARTESIAN_POINT ( 'NONE',  ( -0.8256784875976853622, -7.476520917080001105, -434.9497249379059554 ) ) ;
#7965=CARTESIAN_POINT ( 'NONE',  ( -1.534682465043628152, -2.530859607614999174, -434.5877046317544909 ) ) ;
#7973=DIRECTION ( 'NONE',  ( 0.7220286942758216142, 0.000000000000000000, 0.6918631112021741414 ) ) ;
#7980=ORIENTED_EDGE ( 'NONE', *, *, #5420, .F. ) ;
#7989=( GEOMETRIC_REPRESENTATION_CONTEXT ( 3 ) GLOBAL_UNCERTAINTY_ASSIGNED_CONTEXT ( ( #6025 ) ) GLOBAL_UNIT_ASSIGNED_CONTEXT ( ( #8367, #1821, #208 ) ) REPRESENTATION_CONTEXT ( 'NONE', 'WORKASPACE' ) );
#7991=LINE ( 'NONE', #629, #6523 ) ;
#7995=ORIENTED_EDGE ( 'NONE', *, *, #8075, .F. ) ;
#8006=ORIENTED_EDGE ( 'NONE', *, *, #7014, .F. ) ;
#8017=CARTESIAN_POINT ( 'NONE',  ( -0.9555993562026697807, -2.504535365192000373, -434.3261081466394558 ) ) ;
#8018=ORIENTED_EDGE ( 'NONE', *, *, #3459, .F. ) ;
#8023=CARTESIAN_POINT ( 'NONE',  ( -0.6467809861380701131, -2.500001317010999813, -434.1465151195269527 ) ) ;
#8027=ADVANCED_FACE ( 'NONE', ( #7474 ), #8220, .F. ) ;
#8047=ADVANCED_FACE ( 'NONE', ( #3500 ), #167, .F. ) ;
#8050=DIRECTION ( 'NONE',  ( 0.1283609399493171321, -0.9912279006826364425, 0.03147567320362415488 ) ) ;
#8051=CARTESIAN_POINT ( 'NONE',  ( -14.98500449093754483, -3.491150269972000064, -438.4247239981262396 ) ) ;
#8070=CARTESIAN_POINT ( 'NONE',  ( -0.7259853328840938369, -2.547408842041999133, -434.4258892964173242 ) ) ;
#8075=EDGE_CURVE ( 'NONE', #4227, #10390, #326, .T. ) ;
#8077=UNCERTAINTY_MEASURE_WITH_UNIT (LENGTH_MEASURE( 1.000000000000000082E-05 ), #5105, 'distance_accuracy_value', 'NONE');
#8082=ORIENTED_EDGE ( 'NONE', *, *, #9520, .T. ) ;
#8092=ORIENTED_EDGE ( 'NONE', *, *, #5002, .T. ) ;
#8094=CARTESIAN_POINT ( 'NONE',  ( -9.379635717049819021, -3.022673432387137815, -437.0255164798005012 ) ) ;
#8096=VECTOR ( 'NONE', #8914, 1000.000000000000114 ) ;
#8113=VERTEX_POINT ( 'NONE', #6989 ) ;
#8122=CARTESIAN_POINT ( 'NONE',  ( -4.742836899564842668, -6.886698231682709448, -436.5235822008777973 ) ) ;
#8132=CARTESIAN_POINT ( 'NONE',  ( -16.17578790646000186, -2.500000000000000000, -433.5685902625999688 ) ) ;
#8133=CARTESIAN_POINT ( 'NONE',  ( -0.7111276526388954355, -7.454525072244997830, -434.4156653599139304 ) ) ;
#8139=ORIENTED_EDGE ( 'NONE', *, *, #5745, .T. ) ;
#8140=CYLINDRICAL_SURFACE ( 'NONE', #1592, 3.500000000000006217 ) ;
#8177=CARTESIAN_POINT ( 'NONE',  ( -3.729767414393887481, -7.030426507993915664, -436.1287081606701008 ) ) ;
#8178=CARTESIAN_POINT ( 'NONE',  ( -14.92545173715291007, -5.838463984847977351, -438.6675860777683056 ) ) ;
#8180=CYLINDRICAL_SURFACE ( 'NONE', #8314, 0.9999999999999971134 ) ;
#8182=CARTESIAN_POINT ( 'NONE',  ( -1.582650547086741799, -7.339339277715000165, -435.1382983596024019 ) ) ;
#8185=CARTESIAN_POINT ( 'NONE',  ( -0.4974408136799305380, -7.489648966280001652, -434.5175391694793916 ) ) ;
#8193=VERTEX_POINT ( 'NONE', #2304 ) ;
#8197=CARTESIAN_POINT ( 'NONE',  ( -2.971126855877241013, -7.358725049446134037, -435.1576531919852755 ) ) ;
#8204=CIRCLE ( 'NONE', #9069, 3.500000000000005773 ) ;
#8220=PLANE ( 'NONE',  #4301 ) ;
#8222=CARTESIAN_POINT ( 'NONE',  ( -0.6597201369859407860, -2.500000714168999938, -434.1397697187372273 ) ) ;
#8232=CARTESIAN_POINT ( 'NONE',  ( -0.2899903387719476311, -7.542418068424997735, -434.1586100945300473 ) ) ;
#8235=VERTEX_POINT ( 'NONE', #9774 ) ;
#8278=CARTESIAN_POINT ( 'NONE',  ( -14.96085924495833375, -6.066301387037711379, -438.5231907234968958 ) ) ;
#8284=CARTESIAN_POINT ( 'NONE',  ( -1.076134953867535549, -7.413975726001998723, -434.6066135568960362 ) ) ;
#8310=DIRECTION ( 'NONE',  ( 0.9627073223221466192, 0.1321616141473069550, 0.2360676159351401404 ) ) ;
#8314=AXIS2_PLACEMENT_3D ( 'NONE', #815, #6173, #2099 ) ;
#8328=CARTESIAN_POINT ( 'NONE',  ( -1.418770314803618815, -2.864400061963000788, -435.1301057596324995 ) ) ;
#8332=CARTESIAN_POINT ( 'NONE',  ( -1.166138655389787004, -2.532879817436650693, -434.4904125972011570 ) ) ;
#8334=CARTESIAN_POINT ( 'NONE',  ( -2.575131942425901599, -6.981554778721000609, -435.4819513718353505 ) ) ;
#8336=CARTESIAN_POINT ( 'NONE',  ( -0.1338654248474115960, -2.334823577025999075, -433.9583966923889875 ) ) ;
#8367=( LENGTH_UNIT ( ) NAMED_UNIT ( * ) SI_UNIT ( .MILLI., .METRE. ) );
#8377=EDGE_CURVE ( 'NONE', #5498, #78, #7991, .T. ) ;
#8379=CARTESIAN_POINT ( 'NONE',  ( -8.042176964449417653, -2.829147761587998744, -436.6151782268157717 ) ) ;
#8385=CARTESIAN_POINT ( 'NONE',  ( -5.273242226636224217, -7.500000000000000000, -350.0814130718403590 ) ) ;
#8388=FACE_OUTER_BOUND ( 'NONE', #5469, .T. ) ;
#8392=CARTESIAN_POINT ( 'NONE',  ( 8.385892640053510760, -5.754955315852783748, -525.7042111492452250 ) ) ;
#8404=CARTESIAN_POINT ( 'NONE',  ( -14.98500449093754483, -6.508849730028000380, -438.4247239981262396 ) ) ;
#8417=AXIS2_PLACEMENT_3D ( 'NONE', #7582, #8577, #1222 ) ;
#8429=DIRECTION ( 'NONE',  ( -0.9712267471052612455, 0.000000000000000000, -0.2381566831044910626 ) ) ;
#8434=CARTESIAN_POINT ( 'NONE',  ( -6.057194280361955840, -7.279247941943998157, -436.0403555669980733 ) ) ;
#8440=CARTESIAN_POINT ( 'NONE',  ( 9.297655439795304844, -5.886997446105330489, -525.2645627975454090 ) ) ;
#8461=ORIENTED_EDGE ( 'NONE', *, *, #7591, .F. ) ;
#8467=CARTESIAN_POINT ( 'NONE',  ( -0.8419518381993236211, -7.499550864176998566, -434.2611549955821033 ) ) ;
#8469=AXIS2_PLACEMENT_3D ( 'NONE', #4918, #3203, #8947 ) ;
#8486=CARTESIAN_POINT ( 'NONE',  ( -1.582652182125599660, -2.660653890702000091, -435.1382991101020821 ) ) ;
#8489=CARTESIAN_POINT ( 'NONE',  ( -13.35722247976206312, -6.863431602888001137, -438.0342774710397862 ) ) ;
#8495=B_SPLINE_CURVE_WITH_KNOTS ( 'NONE', 3,
 ( #1473, #4754, #2440, #5710, #824, #8023, #6574 ),
 .UNSPECIFIED., .F., .F.,
 ( 4, 1, 1, 1, 4 ),
 ( 0.000000000000000000, 0.2500000000000000000, 0.5000000000000000000, 0.7500000000000000000, 1.000000000000000000 ),
 .UNSPECIFIED. ) ;
#8496=CARTESIAN_POINT ( 'NONE',  ( -1.551408298843238054, -7.347010659421000511, -435.2528021670048020 ) ) ;
#8520=CARTESIAN_POINT ( 'NONE',  ( -0.7493775555037957004, -7.501813285185003011, -434.1959393140418797 ) ) ;
#8534=CARTESIAN_POINT ( 'NONE',  ( -2.081727251769323050, -2.733745693750686989, -435.4229215395205301 ) ) ;
#8536=CARTESIAN_POINT ( 'NONE',  ( -9.896141615135300995, -5.985941516016800357, -437.8432809189114892 ) ) ;
#8539=DIRECTION ( 'NONE',  ( -0.000000000000000000, 1.000000000000000000, 0.000000000000000000 ) ) ;
#8566=CARTESIAN_POINT ( 'NONE',  ( -0.5973619912582514013, -7.470029452637001022, -434.3275123593290914 ) ) ;
#8577=DIRECTION ( 'NONE',  ( 0.000000000000000000, -1.000000000000000000, 0.000000000000000000 ) ) ;
#8578=DIRECTION ( 'NONE',  ( -0.9712267471052594692, 0.000000000000000000, -0.2381566831044984178 ) ) ;
#8606=ORIENTED_EDGE ( 'NONE', *, *, #5460, .F. ) ;
#8608=FACE_OUTER_BOUND ( 'NONE', #2737, .T. ) ;
#8627=CARTESIAN_POINT ( 'NONE',  ( -1.170813146951170225, -7.466834095521711845, -434.4923879807246294 ) ) ;
#8629=DIRECTION ( 'NONE',  ( 0.9627072927120896573, 0.1321637200909031584, 0.2360665576711206692 ) ) ;
#8634=CARTESIAN_POINT ( 'NONE',  ( 0.000000000000000000, 0.000000000000000000, 0.000000000000000000 ) ) ;
#8638=CARTESIAN_POINT ( 'NONE',  ( -0.6524225759890166509, -2.520141586570888492, -434.5249754051499167 ) ) ;
#8641=CARTESIAN_POINT ( 'NONE',  ( -7.666814856007332146, -6.251400993695000352, -437.4143429429252592 ) ) ;
#8700=CARTESIAN_POINT ( 'NONE',  ( -1.658528026434172631, -7.334393795902656166, -435.0029499069592589 ) ) ;
#8709=CARTESIAN_POINT ( 'NONE',  ( -0.4971732199403511299, -2.511415353335999967, -434.1478469224045966 ) ) ;
#8716=VERTEX_POINT ( 'NONE', #3282 ) ;
#8727=CARTESIAN_POINT ( 'NONE',  ( -0.5929282851181935099, -7.526005961551003764, -434.8233273616743872 ) ) ;
#8733=CARTESIAN_POINT ( 'NONE',  ( -6.514686351705899270, -2.852628117829832277, -436.2336205443476729 ) ) ;
#8736=CARTESIAN_POINT ( 'NONE',  ( -1.813125098999968543, -7.427867185880000278, -434.7536662776001322 ) ) ;
#8746=CARTESIAN_POINT ( 'NONE',  ( -14.92529112109648004, -4.159649519892460567, -438.6682410860930759 ) ) ;
#8765=CARTESIAN_POINT ( 'NONE',  ( -1.419469786162590674, -2.618831809747000694, -434.7498648015279059 ) ) ;
#8772=CARTESIAN_POINT ( 'NONE',  ( -15.16362200326591569, -2.500000000000000000, -437.6963039377973246 ) ) ;
#8781=AXIS2_PLACEMENT_3D ( 'NONE', #2952, #5416, #1391 ) ;
#8788=CARTESIAN_POINT ( 'NONE',  ( -5.561800649038728395, -2.795979873486618139, -435.9619414120115266 ) ) ;
#8814=( BOUNDED_SURFACE ( )  B_SPLINE_SURFACE ( 3, 3, ( 
 ( #5536, #2326, #10484, #1518, #7965, #5486, #8820, #4747, #7161, #6346, #8017, #3020, #2968, #7856, #4689, #3126, #3184, #1406, #6239, #5594 ),
 ( #611, #3884, #8876, #550, #8765, #5431, #4798, #9738, #10327, #1352, #2380, #8070, #1300, #1466, #5644, #10432, #8709, #4580, #501, #714 ),
 ( #3072, #3769, #3987, #660, #9628, #2270, #7062, #3936, #9525, #6457, #7112, #10380, #7269, #2165, #4634, #7905, #6294, #9579, #2218, #7216 ),
 ( #6404, #7323, #1626, #4046, #9147, #10594, #3236, #4851, #9794, #7373, #2537, #7481, #9095, #10007, #4261, #176, #4095, #8336, #1785, #5804 ) ),
 .UNSPECIFIED., .F., .F., .F. ) 
 B_SPLINE_SURFACE_WITH_KNOTS ( ( 4, 4 ),
 ( 4, 1, 1, 1, 1, 1, 1, 1, 1, 1, 1, 1, 1, 1, 1, 1, 1, 4 ),
 ( 0.000000000000000000, 1.000000000000000000 ),
 ( 0.1929541978887999998, 0.2554811723075999796, 0.3278331352657999909, 0.3941678789460000276, 0.4549425011739000047, 0.5106931027059999906, 0.5620016754668999415, 0.6094703044461000641, 0.6536430579613999869, 0.6948991896359000275, 0.7334433934487000206, 0.7692443867375999833, 0.8015803013500999441, 0.8300487060171000131, 0.8556850663905000154, 0.8806332672557000141, 0.9057989055234000331, 0.9210247255515999765 ),
 .UNSPECIFIED. ) 
 GEOMETRIC_REPRESENTATION_ITEM ( )  RATIONAL_B_SPLINE_SURFACE ( (
 ( 1.026139272308000061, 1.026139272308000061, 1.026139272308000061, 1.026139272308000061, 1.026139272308000061, 1.026139272308000061, 1.026139272308000061, 1.026139272308000061, 1.026139272308000061, 1.026139272308000061, 1.026139272308000061, 1.026139272308000061, 1.026139272308000061, 1.026139272308000061, 1.026139272308000061, 1.026139272308000061, 1.026139272308000061, 1.026139272308000061, 1.026139272308000061, 1.026139272308000061),
 ( 0.9912869092307000640, 0.9912869092307000640, 0.9912869092307000640, 0.9912869092307000640, 0.9912869092307000640, 0.9912869092307000640, 0.9912869092307000640, 0.9912869092307000640, 0.9912869092307000640, 0.9912869092307000640, 0.9912869092307000640, 0.9912869092307000640, 0.9912869092307000640, 0.9912869092307000640, 0.9912869092307000640, 0.9912869092307000640, 0.9912869092307000640, 0.9912869092307000640, 0.9912869092307000640, 0.9912869092307000640),
 ( 0.9912869092307000640, 0.9912869092307000640, 0.9912869092307000640, 0.9912869092307000640, 0.9912869092307000640, 0.9912869092307000640, 0.9912869092307000640, 0.9912869092307000640, 0.9912869092307000640, 0.9912869092307000640, 0.9912869092307000640, 0.9912869092307000640, 0.9912869092307000640, 0.9912869092307000640, 0.9912869092307000640, 0.9912869092307000640, 0.9912869092307000640, 0.9912869092307000640, 0.9912869092307000640, 0.9912869092307000640),
 ( 1.026139272308000061, 1.026139272308000061, 1.026139272308000061, 1.026139272308000061, 1.026139272308000061, 1.026139272308000061, 1.026139272308000061, 1.026139272308000061, 1.026139272308000061, 1.026139272308000061, 1.026139272308000061, 1.026139272308000061, 1.026139272308000061, 1.026139272308000061, 1.026139272308000061, 1.026139272308000061, 1.026139272308000061, 1.026139272308000061, 1.026139272308000061, 1.026139272308000061) ) ) 
 REPRESENTATION_ITEM ( '' )  SURFACE ( )  );
#8820=CARTESIAN_POINT ( 'NONE',  ( -1.302538776795788555, -2.519749681487999382, -434.4904071209729182 ) ) ;
#8842=CARTESIAN_POINT ( 'NONE',  ( 3.875825478601963248, -2.500000000000000000, -431.3627451401119970 ) ) ;
#8860=CARTESIAN_POINT ( 'NONE',  ( -14.90555606507826170, -4.246020682187605644, -438.7487226161961189 ) ) ;
#8862=ORIENTED_EDGE ( 'NONE', *, *, #1682, .F. ) ;
#8876=CARTESIAN_POINT ( 'NONE',  ( -1.698905183273398123, -2.643595541597000942, -434.8557611820924080 ) ) ;
#8895=CARTESIAN_POINT ( 'NONE',  ( 28.53863984632670636, -2.500000000000000000, -506.8274460463252353 ) ) ;
#8901=CARTESIAN_POINT ( 'NONE',  ( -11.30134585255874313, -3.136348707664786239, -437.5214317848546557 ) ) ;
#8906=EDGE_CURVE ( 'NONE', #8235, #4938, #5051, .T. ) ;
#8914=DIRECTION ( 'NONE',  ( -0.9712267471052600243, 4.782300904073985984E-08, -0.2381566831044907573 ) ) ;
#8935=FACE_OUTER_BOUND ( 'NONE', #10511, .T. ) ;
#8936=CARTESIAN_POINT ( 'NONE',  ( -1.713290296832884474, -7.307229827337997641, -435.0847711425938087 ) ) ;
#8937=MANIFOLD_SOLID_BREP ( 'Stock-MAS-686-1', #1450 ) ;
#8947=DIRECTION ( 'NONE',  ( 0.9712267471052594692, 0.000000000000000000, 0.2381566831044984456 ) ) ;
#8976=AXIS2_PLACEMENT_3D ( 'NONE', #6246, #5438, #7973 ) ;
#8985=CARTESIAN_POINT ( 'NONE',  ( -3.554202447527484487, -7.055426064859528168, -436.0573967677022438 ) ) ;
#8992=DIRECTION ( 'NONE',  ( 0.000000000000000000, -1.000000000000000000, 0.000000000000000000 ) ) ;
#8994=CARTESIAN_POINT ( 'NONE',  ( -0.2029048030085919552, -7.657414115644002983, -433.8324684254904469 ) ) ;
#9000=ORIENTED_EDGE ( 'NONE', *, *, #6063, .T. ) ;
#9001=CARTESIAN_POINT ( 'NONE',  ( -0.6596894340221253206, -7.499999891561000886, -434.1397621899948263 ) ) ;
#9010=CARTESIAN_POINT ( 'NONE',  ( -2.272374192480355326, -7.400653393618207510, -434.9211848868894208 ) ) ;
#9037=CARTESIAN_POINT ( 'NONE',  ( -1.832041979401632714, -7.303110144047968433, -435.2805036650163970 ) ) ;
#9039=CARTESIAN_POINT ( 'NONE',  ( -14.95234154667176973, -5.997675161540820810, -438.5579267480833323 ) ) ;
#9045=VERTEX_POINT ( 'NONE', #4673 ) ;
#9048=CARTESIAN_POINT ( 'NONE',  ( -1.652955156006773230, -7.314598583700001377, -435.0632706482025469 ) ) ;
#9051=ORIENTED_EDGE ( 'NONE', *, *, #5619, .T. ) ;
#9053=ORIENTED_EDGE ( 'NONE', *, *, #9566, .F. ) ;
#9055=ORIENTED_EDGE ( 'NONE', *, *, #6395, .T. ) ;
#9065=CARTESIAN_POINT ( 'NONE',  ( -13.22841524816015202, -3.249999927714000147, -437.9939944912570127 ) ) ;
#9069=AXIS2_PLACEMENT_3D ( 'NONE', #3511, #283, #5219 ) ;
#9084=CARTESIAN_POINT ( 'NONE',  ( -1.761667614806367244, -2.511152837933000370, -434.6216513933122769 ) ) ;
#9090=AXIS2_PLACEMENT_3D ( 'NONE', #3293, #7330, #1582 ) ;
#9091=CARTESIAN_POINT ( 'NONE',  ( -1.073657119321965059, -2.527164246181165197, -434.4475771139335052 ) ) ;
#9095=CARTESIAN_POINT ( 'NONE',  ( -0.3336219746636178707, -2.411421344994997717, -434.6316404192452865 ) ) ;
#9098=VECTOR ( 'NONE', #483, 1000.000000000000000 ) ;
#9100=CARTESIAN_POINT ( 'NONE',  ( 6.710635551220206274, -4.448381107550146929, -525.2761360244785465 ) ) ;
#9102=CARTESIAN_POINT ( 'NONE',  ( -0.3470087687485771677, -7.585217605017000153, -434.6423010044687203 ) ) ;
#9116=CARTESIAN_POINT ( 'NONE',  ( -11.30134943970389827, -6.863654245155042410, -437.5214327350141730 ) ) ;
#9136=VERTEX_POINT ( 'NONE', #6224 ) ;
#9137=CARTESIAN_POINT ( 'NONE',  ( -13.28926728532226242, -3.829332416735001576, -437.9231028215058359 ) ) ;
#9144=CARTESIAN_POINT ( 'NONE',  ( -1.419234048971399931, -7.135492406320001813, -435.1303133261055223 ) ) ;
#9147=CARTESIAN_POINT ( 'NONE',  ( -1.193878590405294648, -2.592889965380001716, -435.1143622073087158 ) ) ;
#9152=CARTESIAN_POINT ( 'NONE',  ( -1.449792573629281600, -7.363504377864001249, -435.2149157260363381 ) ) ;
#9169=( BOUNDED_CURVE ( )  B_SPLINE_CURVE ( 3, ( #418, #2892, #7091, #3646, #4607, #1987, #5352, #6929, #2844, #4498, #3698, #6160, #7881, #10356, #7035, #9549, #2190, #8627, #1274, #2995, #4663, #10306, #6270, #5458, #475, #8736 ),
 .UNSPECIFIED., .F., .F. ) 
 B_SPLINE_CURVE_WITH_KNOTS ( ( 4, 1, 1, 1, 1, 1, 1, 1, 1, 1, 1, 1, 1, 1, 1, 1, 1, 1, 1, 1, 1, 1, 1, 4 ),
 ( 0.000000000000000000, 0.006575387376420720360, 0.03147587580142015284, 0.05343946111830009255, 0.07456689176594544222, 0.09618900060869983726, 0.1191358387887401504, 0.1441625736054258922, 0.1719175949757547894, 0.2028430032774542480, 0.2370252242332172854, 0.2743986122632974256, 0.3149466209281155393, 0.3587386281848603531, 0.4061912593601564314, 0.4578269296042451475, 0.5140479793078506221, 0.5747700779972666485, 0.6397184740335285502, 0.7086229277996399789, 0.7817513793272220513, 0.8601134552957673263, 0.9447709961445381888, 1.000000000000000000 ),
 .UNSPECIFIED. ) 
 CURVE ( )  GEOMETRIC_REPRESENTATION_ITEM ( )  RATIONAL_B_SPLINE_CURVE ( ( 1.017162749436847813, 1.017162749436847813, 1.017162749436847813, 1.017162749436847813, 1.017162749436847813, 1.017162749436847813, 1.017162749436847813, 1.017162749436847813, 1.017162749436847813, 1.017162749436847813, 1.017162749436847813, 1.017162749436847813, 1.017162749436847813, 1.017162749436847813, 1.017162749436847813, 1.017162749436847813, 1.017162749436847813, 1.017162749436847813, 1.017162749436847813, 1.017162749436847813, 1.017162749436847813, 1.017162749436847813, 1.017162749436847813, 1.017162749436847813, 1.017162749436847813, 1.017162749436847813 ) ) 
 REPRESENTATION_ITEM ( '' )  );
#9192=VERTEX_POINT ( 'NONE', #10580 ) ;
#9194=AXIS2_PLACEMENT_3D ( 'NONE', #4478, #2771, #2722 ) ;
#9205=CARTESIAN_POINT ( 'NONE',  ( -13.01014152926537548, -6.185120192877000989, -437.8675655776580129 ) ) ;
#9229=ORIENTED_EDGE ( 'NONE', *, *, #7014, .T. ) ;
#9248=CARTESIAN_POINT ( 'NONE',  ( -1.813125407131493949, -2.572135581867000198, -434.7536649739391237 ) ) ;
#9259=CARTESIAN_POINT ( 'NONE',  ( -2.038881997165930215, -7.478227285005997871, -434.7312091017502667 ) ) ;
#9263=CARTESIAN_POINT ( 'NONE',  ( 7.083228393897874398, -4.408350100845710884, -525.5349554852709844 ) ) ;
#9265=VECTOR ( 'NONE', #10005, 1000.000000000000114 ) ;
#9271=VERTEX_POINT ( 'NONE', #3195 ) ;
#9292=CARTESIAN_POINT ( 'NONE',  ( -0.5403494531946965163, -7.486475365814998284, -434.0354456928992022 ) ) ;
#9293=SURFACE_STYLE_USAGE ( .BOTH. , #6818 ) ;
#9315=CARTESIAN_POINT ( 'NONE',  ( 6.052780067456072999, -5.500000000000000000, -524.2189112390747141 ) ) ;
#9342=( NAMED_UNIT ( * ) PLANE_ANGLE_UNIT ( ) SI_UNIT ( $, .RADIAN. ) );
#9358=VECTOR ( 'NONE', #4008, 1000.000000000000114 ) ;
#9362=DIRECTION ( 'NONE',  ( 0.000000000000000000, -1.000000000000000000, 0.000000000000000000 ) ) ;
#9369=CARTESIAN_POINT ( 'NONE',  ( 8.355542331113237964, -5.750853016826391162, -525.7099095707894776 ) ) ;
#9382=DIRECTION ( 'NONE',  ( -0.1124491875265152124, 0.000000000000000000, 0.9936574763089273121 ) ) ;
#9391=EDGE_CURVE ( 'NONE', #5334, #5915, #435, .T. ) ;
#9392=CARTESIAN_POINT ( 'NONE',  ( -1.554031834198139839, -7.468176060817003581, -434.5954497281065301 ) ) ;
#9403=CIRCLE ( 'NONE', #140, 0.7500000000000247580 ) ;
#9404=DIRECTION ( 'NONE',  ( -0.2381566825879641303, -3.988721798185001137E-09, 0.9712267472319199291 ) ) ;
#9407=CARTESIAN_POINT ( 'NONE',  ( -8.155631454398118763, -3.591146263826743290, -437.6540831751978544 ) ) ;
#9419=ORIENTED_EDGE ( 'NONE', *, *, #1759, .T. ) ;
#9421=CARTESIAN_POINT ( 'NONE',  ( -0.5535498271043974849, -7.499999952522999891, -434.2938920418101816 ) ) ;
#9427=EDGE_CURVE ( 'NONE', #6833, #7332, #7134, .T. ) ;
#9435=ORIENTED_EDGE ( 'NONE', *, *, #5848, .F. ) ;
#9441=CARTESIAN_POINT ( 'NONE',  ( -0.7362249915901031283, -7.501925031340999084, -434.1840766770703226 ) ) ;
#9450=FACE_OUTER_BOUND ( 'NONE', #5021, .T. ) ;
#9478=LINE ( 'NONE', #6094, #4687 ) ;
#9489=CARTESIAN_POINT ( 'NONE',  ( -0.7659865709275307522, -7.501556614171002835, -434.2093659254040858 ) ) ;
#9518=VECTOR ( 'NONE', #327, 1000.000000000000000 ) ;
#9520=EDGE_CURVE ( 'NONE', #2925, #78, #3348, .T. ) ;
#9525=CARTESIAN_POINT ( 'NONE',  ( -0.8363673731450661508, -2.571798426227997592, -434.7280016174766502 ) ) ;
#9535=VERTEX_POINT ( 'NONE', #7399 ) ;
#9541=CARTESIAN_POINT ( 'NONE',  ( -0.3010101818115299976, -7.537189068435002248, -434.2310189891967411 ) ) ;
#9549=CARTESIAN_POINT ( 'NONE',  ( -1.034036475800059751, -7.475296907637412502, -434.4283210023707511 ) ) ;
#9566=EDGE_CURVE ( 'NONE', #4172, #6718, #1110, .T. ) ;
#9569=CARTESIAN_POINT ( 'NONE',  ( 1.525345003100600394, -7.500000000000000000, -348.4143162901089568 ) ) ;
#9578=CARTESIAN_POINT ( 'NONE',  ( -0.9958895184599025896, -7.426437712707262051, -434.8066008177434583 ) ) ;
#9579=CARTESIAN_POINT ( 'NONE',  ( -0.3079143655542058711, -2.454520757324000435, -434.0165891553489814 ) ) ;
#9611=AXIS2_PLACEMENT_3D ( 'NONE', #3444, #3552, #6780 ) ;
#9615=LINE ( 'NONE', #3111, #7079 ) ;
#9621=CARTESIAN_POINT ( 'NONE',  ( -1.813125098999968543, -7.427867185880000278, -434.7536662776001322 ) ) ;
#9628=CARTESIAN_POINT ( 'NONE',  ( -1.301874420428522861, -2.640235564664999757, -434.9315895259924218 ) ) ;
#9631=CARTESIAN_POINT ( 'NONE',  ( -14.37110465573396212, -2.500000000000000000, -348.9812360766022721 ) ) ;
#9641=VERTEX_POINT ( 'NONE', #1310 ) ;
#9654=CARTESIAN_POINT ( 'NONE',  ( -14.37110465573396212, -7.500000000000000000, -348.9812360766022721 ) ) ;
#9667=ORIENTED_EDGE ( 'NONE', *, *, #1338, .T. ) ;
#9668=CARTESIAN_POINT ( 'NONE',  ( 9.378959784071181360, -4.100000000000000533, -525.1866552614185366 ) ) ;
#9676=PRODUCT_CONTEXT ( 'NONE', #4147, 'mechanical' ) ;
#9683=CARTESIAN_POINT ( 'NONE',  ( -0.5535498271043974849, -7.499999952522999891, -434.2938920418101816 ) ) ;
#9684=FACE_OUTER_BOUND ( 'NONE', #5453, .T. ) ;
#9687=DIRECTION ( 'NONE',  ( -0.9627070496199739980, 0.1321637200910051047, -0.2360675490272045873 ) ) ;
#9705=ADVANCED_FACE ( 'NONE', ( #8608 ), #1968, .T. ) ;
#9707=( GEOMETRIC_REPRESENTATION_CONTEXT ( 3 ) GLOBAL_UNCERTAINTY_ASSIGNED_CONTEXT ( ( #2278 ) ) GLOBAL_UNIT_ASSIGNED_CONTEXT ( ( #10040, #9342, #2682 ) ) REPRESENTATION_CONTEXT ( 'NONE', 'WORKASPACE' ) );
#9718=EDGE_CURVE ( 'NONE', #8716, #7492, #601, .T. ) ;
#9723=DIRECTION ( 'NONE',  ( 0.7220286942758216142, 0.000000000000000000, 0.6918631112021741414 ) ) ;
#9738=CARTESIAN_POINT ( 'NONE',  ( -1.071307256257647333, -2.585569669607997945, -434.6046133433468412 ) ) ;
#9745=CARTESIAN_POINT ( 'NONE',  ( -0.3590672782033171861, -7.540140950748998705, -433.9280555215146364 ) ) ;
#9758=DIRECTION ( 'NONE',  ( -0.2381566831044910626, 0.000000000000000000, 0.9712267471052612455 ) ) ;
#9774=CARTESIAN_POINT ( 'NONE',  ( 10.54676984209158519, -2.500000000000000000, -347.8422498368975084 ) ) ;
#9779=LINE ( 'NONE', #7311, #6202 ) ;
#9791=DIRECTION ( 'NONE',  ( 0.7172627762233165782, 0.1147078669353000374, 0.6872963080852203532 ) ) ;
#9794=CARTESIAN_POINT ( 'NONE',  ( -0.7127201389310124924, -2.500198451567999580, -434.8920403824821506 ) ) ;
#9795=CARTESIAN_POINT ( 'NONE',  ( 1.525345003100600394, -7.500000000000000000, -348.4143162901089568 ) ) ;
#9797=VECTOR ( 'NONE', #4722, 1000.000000000000000 ) ;
#9801=CARTESIAN_POINT ( 'NONE',  ( -0.7425212270488497079, -7.493595516397002498, -434.9074498605589838 ) ) ;
#9818=CIRCLE ( 'NONE', #4839, 12.50000000000000178 ) ;
#9839=CARTESIAN_POINT ( 'NONE',  ( -15.16362200326591569, -6.750000000000000000, -437.6963039377973246 ) ) ;
#9846=CARTESIAN_POINT ( 'NONE',  ( -14.89424055888783727, -5.714488051281095160, -438.7948683809335080 ) ) ;
#9855=CARTESIAN_POINT ( 'NONE',  ( -0.7911908081797823789, -7.435692558170999611, -434.7046119063388119 ) ) ;
#9861=ORIENTED_EDGE ( 'NONE', *, *, #5460, .T. ) ;
#9874=DIRECTION ( 'NONE',  ( -0.9712267471052612455, 0.000000000000000000, -0.2381566831044910626 ) ) ;
#9893=CARTESIAN_POINT ( 'NONE',  ( -2.852327370720492805, -2.558519736919000032, -435.0254095138128605 ) ) ;
#9894=LINE ( 'NONE', #1435, #9797 ) ;
#9905=FACE_BOUND ( 'NONE', #253, .T. ) ;
#9906=CARTESIAN_POINT ( 'NONE',  ( -1.821036076062871656, -7.345996400954998506, -434.8999269110483397 ) ) ;
#9909=ORIENTED_EDGE ( 'NONE', *, *, #1952, .T. ) ;
#9916=DIRECTION ( 'NONE',  ( -0.1124491875265153235, 0.000000000000000000, 0.9936574763089273121 ) ) ;
#9917=VECTOR ( 'NONE', #6932, 1000.000000000000000 ) ;
#9918=CARTESIAN_POINT ( 'NONE',  ( -6.514701929829219473, -7.147380552937434572, -436.2336181546095872 ) ) ;
#9929=CARTESIAN_POINT ( 'NONE',  ( -14.74684780783305449, -4.500000000000000888, -439.3959507452315165 ) ) ;
#9941=CARTESIAN_POINT ( 'NONE',  ( -7.669357409124427427, -3.748921511560000752, -437.4148671000394302 ) ) ;
#9947=CARTESIAN_POINT ( 'NONE',  ( -1.803054005006139882, -2.571757231099727647, -434.7497522307571103 ) ) ;
#9949=( NAMED_UNIT ( * ) SI_UNIT ( $, .STERADIAN. ) SOLID_ANGLE_UNIT ( ) );
#9950=CARTESIAN_POINT ( 'NONE',  ( -2.852011294728740154, -7.441500538535999354, -435.0252681240257857 ) ) ;
#9958=CARTESIAN_POINT ( 'NONE',  ( 8.327676564211852650, -5.747092138782196713, -525.7147768702978965 ) ) ;
#9975=CARTESIAN_POINT ( 'NONE',  ( -0.5535498271043974849, -7.499999952522999891, -434.2938920418101816 ) ) ;
#9996=CARTESIAN_POINT ( 'NONE',  ( -4.264364113041657411, -2.626784553234001063, -435.4922059969647421 ) ) ;
#10001=VERTEX_POINT ( 'NONE', #287 ) ;
#10002=CARTESIAN_POINT ( 'NONE',  ( -0.7845517089437358260, -2.508978674445781820, -434.2902902441725814 ) ) ;
#10005=DIRECTION ( 'NONE',  ( 0.7220286942758216142, 0.000000000000000000, 0.6918631112021741414 ) ) ;
#10007=CARTESIAN_POINT ( 'NONE',  ( -0.2521427309798530136, -2.389480942926001106, -434.5434516125882851 ) ) ;
#10011=CARTESIAN_POINT ( 'NONE',  ( 9.178407731729972596, -5.867721822115068875, -525.3673751052774605 ) ) ;
#10013=CARTESIAN_POINT ( 'NONE',  ( -14.74684780783305449, -5.500000000000000000, -439.3959507452315165 ) ) ;
#10035=EDGE_CURVE ( 'NONE', #6305, #574, #9169, .T. ) ;
#10040=( LENGTH_UNIT ( ) NAMED_UNIT ( * ) SI_UNIT ( .MILLI., .METRE. ) );
#10043=LINE ( 'NONE', #5954, #2490 ) ;
#10051=CARTESIAN_POINT ( 'NONE',  ( -12.82747756644705284, -4.303278812719999458, -438.3419432558599738 ) ) ;
#10054=EDGE_LOOP ( 'NONE', ( #1663, #10462 ) ) ;
#10057=CARTESIAN_POINT ( 'NONE',  ( 10.54676984209158519, -2.500000000000000000, -347.8422498368975084 ) ) ;
#10089=CARTESIAN_POINT ( 'NONE',  ( -1.457510205898610467, -7.472866546578002200, -434.5559982538129589 ) ) ;
#10100=CARTESIAN_POINT ( 'NONE',  ( -12.01465775597979935, -3.056837257450998102, -437.6905913349352204 ) ) ;
#10110=CARTESIAN_POINT ( 'NONE',  ( 8.413421927184343119, -4.241283675082794247, -525.6983829592555821 ) ) ;
#10111=VECTOR ( 'NONE', #8629, 999.9999999999998863 ) ;
#10113=CARTESIAN_POINT ( 'NONE',  ( 8.333641625544045084, -5.747896767544797392, -525.7137649939094217 ) ) ;
#10115=ORIENTED_EDGE ( 'NONE', *, *, #342, .T. ) ;
#10119=LINE ( 'NONE', #7800, #44 ) ;
#10144=ORIENTED_EDGE ( 'NONE', *, *, #3063, .F. ) ;
#10155=CARTESIAN_POINT ( 'NONE',  ( -2.240424119748007481, -7.737646341025000041, -436.4485772352342678 ) ) ;
#10178=CARTESIAN_POINT ( 'NONE',  ( -13.22841485905253833, -6.750000122098000155, -437.9939945094035920 ) ) ;
#10185=ORIENTED_EDGE ( 'NONE', *, *, #5677, .F. ) ;
#10194=CARTESIAN_POINT ( 'NONE',  ( -1.073151323001753310, -7.490579005208001462, -434.3854452274036362 ) ) ;
#10197=CARTESIAN_POINT ( 'NONE',  ( 28.53863984632670636, -2.500000000000000000, -506.8274460463252353 ) ) ;
#10221=CYLINDRICAL_SURFACE ( 'NONE', #3028, 19.99999999999999289 ) ;
#10228=EDGE_LOOP ( 'NONE', ( #664, #9861, #840, #4159, #4715, #2656 ) ) ;
#10241=ORIENTED_EDGE ( 'NONE', *, *, #4033, .F. ) ;
#10248=CARTESIAN_POINT ( 'NONE',  ( 1.525345003100600394, -2.500000000000000000, -348.4143162901089568 ) ) ;
#10262=CARTESIAN_POINT ( 'NONE',  ( -0.9955007295007036738, -2.573504618523215104, -434.8063702403939033 ) ) ;
#10289=AXIS2_PLACEMENT_3D ( 'NONE', #9631, #5597, #1521 ) ;
#10299=CARTESIAN_POINT ( 'NONE',  ( -1.941306618757602687, -7.448794727589000075, -434.7455987018001906 ) ) ;
#10306=CARTESIAN_POINT ( 'NONE',  ( -1.522216677011161368, -7.445310505451432803, -434.6409043759791189 ) ) ;
#10307=LINE ( 'NONE', #4664, #10111 ) ;
#10313=CARTESIAN_POINT ( 'NONE',  ( -3.842134514272915524, -2.985559382381202553, -436.1738895293993892 ) ) ;
#10326=CARTESIAN_POINT ( 'NONE',  ( -1.582650547086741799, -7.339339277715000165, -435.1382983596024019 ) ) ;
#10327=CARTESIAN_POINT ( 'NONE',  ( -0.9740888417759976381, -2.575554204550001280, -434.5596432194157615 ) ) ;
#10332=VECTOR ( 'NONE', #2009, 1000.000000000000000 ) ;
#10337=CARTESIAN_POINT ( 'NONE',  ( -6.244201582844205234, -6.675757048814958239, -437.0437999513653153 ) ) ;
#10346=AXIS2_PLACEMENT_3D ( 'NONE', #7306, #8050, #5736 ) ;
#10348=CARTESIAN_POINT ( 'NONE',  ( -0.3480625055678318036, -7.541428400184998715, -433.9440080516719149 ) ) ;
#10355=DIRECTION ( 'NONE',  ( 0.000000000000000000, -1.000000000000000000, 0.000000000000000000 ) ) ;
#10356=CARTESIAN_POINT ( 'NONE',  ( -0.9220120792583293978, -7.482292487583758422, -434.3711255064411603 ) ) ;
#10358=DIRECTION ( 'NONE',  ( -0.000000000000000000, 1.000000000000000000, 0.000000000000000000 ) ) ;
#10380=CARTESIAN_POINT ( 'NONE',  ( -0.5644360195601177965, -2.523842503971001960, -434.5698867567434149 ) ) ;
#10390=VERTEX_POINT ( 'NONE', #1208 ) ;
#10403=CARTESIAN_POINT ( 'NONE',  ( -4.143439832052679961, -2.711403837272623463, -435.5329398554599720 ) ) ;
#10431=CARTESIAN_POINT ( 'NONE',  ( -14.81771799810021584, -5.543961357743112828, -439.1069350289280351 ) ) ;
#10432=CARTESIAN_POINT ( 'NONE',  ( -0.5143507147629048371, -2.516076635578000875, -434.2178808803126913 ) ) ;
#10447=DIRECTION ( 'NONE',  ( -0.9712267471052614676, 0.000000000000000000, -0.2381566831044902022 ) ) ;
#10462=ORIENTED_EDGE ( 'NONE', *, *, #880, .T. ) ;
#10471=DIRECTION ( 'NONE',  ( 0.000000000000000000, -1.000000000000000000, 0.000000000000000000 ) ) ;
#10484=CARTESIAN_POINT ( 'NONE',  ( -1.805690315422955994, -2.544311598584000134, -434.6943802261359338 ) ) ;
#10502=VECTOR ( 'NONE', #10355, 1000.000000000000000 ) ;
#10511=EDGE_LOOP ( 'NONE', ( #5850, #7125, #9909, #1504, #7715, #131, #7663, #7597, #7995, #7437, #9419, #9000 ) ) ;
#10520=CARTESIAN_POINT ( 'NONE',  ( -14.85833869408811125, -4.382513931880057889, -438.9412797724170900 ) ) ;
#10528=EDGE_LOOP ( 'NONE', ( #4326, #2930, #1263, #8082 ) ) ;
#10532=( GEOMETRIC_REPRESENTATION_CONTEXT ( 3 ) GLOBAL_UNCERTAINTY_ASSIGNED_CONTEXT ( ( #8077 ) ) GLOBAL_UNIT_ASSIGNED_CONTEXT ( ( #5105, #1941, #9949 ) ) REPRESENTATION_CONTEXT ( 'NONE', 'WORKASPACE' ) );
#10538=CARTESIAN_POINT ( 'NONE',  ( -3.744595214114432746, -7.028316276732002876, -436.1346940467533955 ) ) ;
#10549=CARTESIAN_POINT ( 'NONE',  ( -0.7589204585291327021, -7.448615989627000999, -434.4456504183515335 ) ) ;
#10551=FACE_OUTER_BOUND ( 'NONE', #5690, .T. ) ;
#10579=CARTESIAN_POINT ( 'NONE',  ( -14.86799266576450584, -4.360433334866828936, -438.9019099114260030 ) ) ;
#10580=CARTESIAN_POINT ( 'NONE',  ( -14.37110465573396212, -2.500000000000000000, -348.9812360766022721 ) ) ;
#10587=SHAPE_DEFINITION_REPRESENTATION ( #1506, #4085 ) ;
#10594=CARTESIAN_POINT ( 'NONE',  ( -1.059650150527880585, -2.568636005655999366, -435.0577782176294477 ) ) ;
#10595=LINE ( 'NONE', #3237, #7457 ) ;
#10598=DIRECTION ( 'NONE',  ( -0.9712267471052612455, -0.000000000000000000, -0.2381566831044910626 ) ) ;
#10599=CARTESIAN_POINT ( 'NONE',  ( -0.1726170993359143480, -7.634036073875003048, -434.4152387547379135 ) ) ;
#10619=CARTESIAN_POINT ( 'NONE',  ( -3.672956643297854651, -2.683304555918673451, -435.3862750469904768 ) ) ;
ENDSEC;
END-ISO-10303-21;
